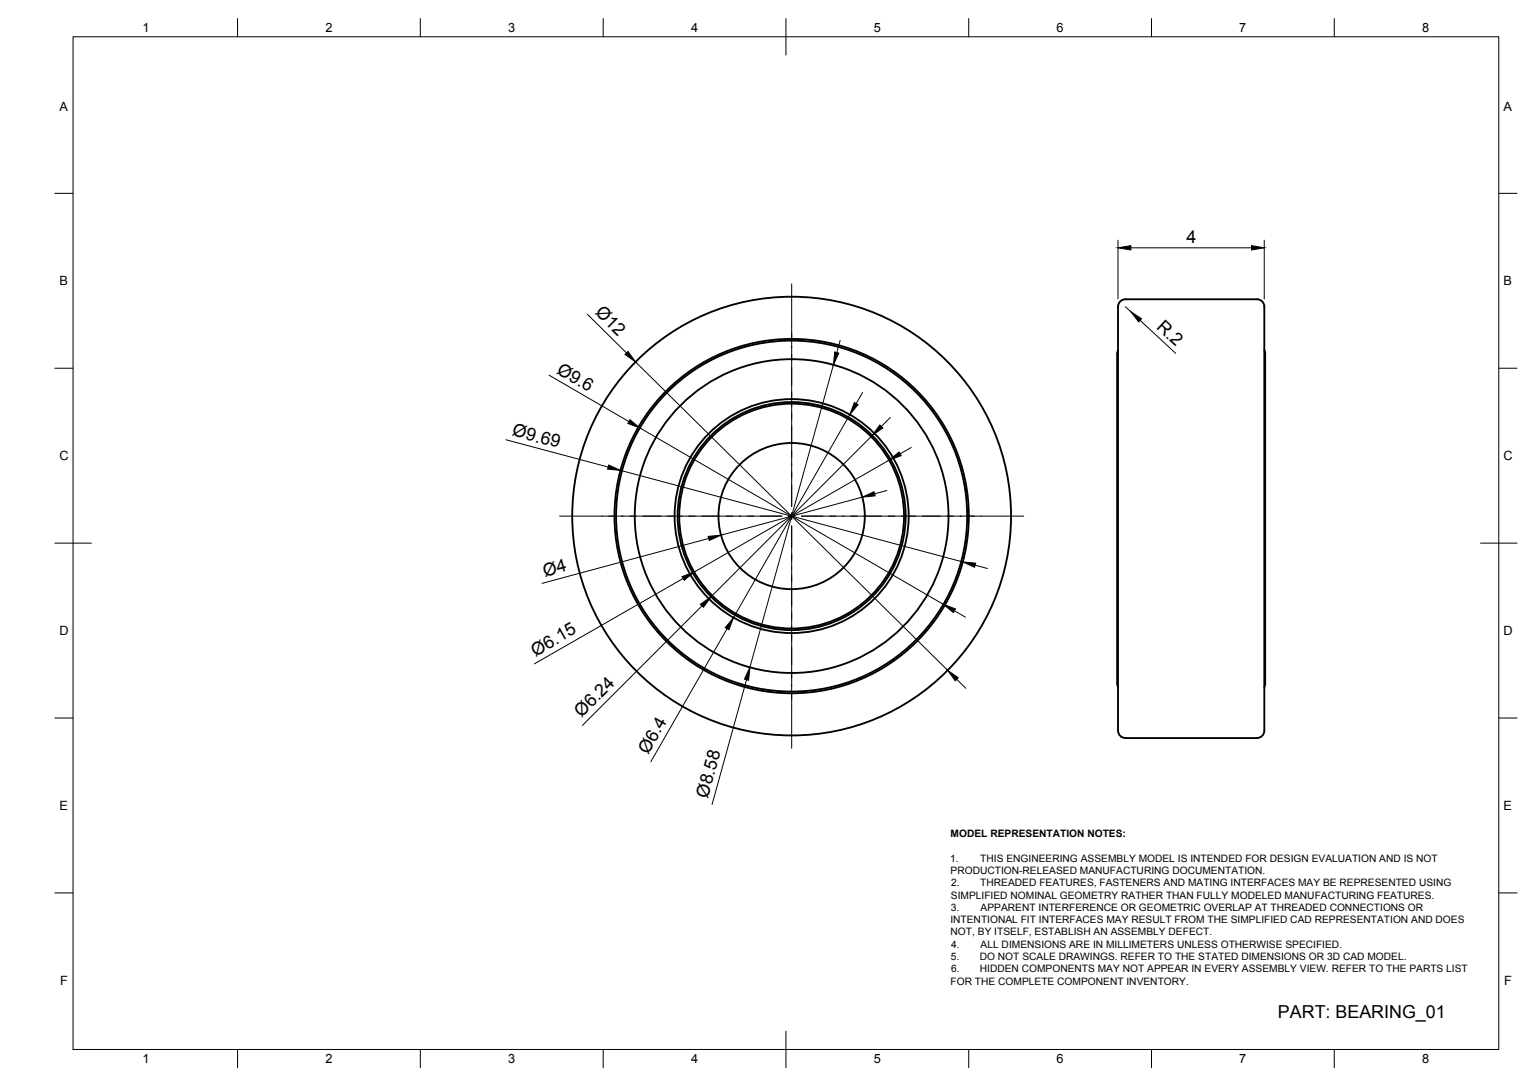
ISO-10303-21;
HEADER;
/* Generated by software containing ST-Developer
 * from STEP Tools, Inc. (www.steptools.com) 
 */

FILE_DESCRIPTION(
/* description */ (''),
/* implementation_level */ '2;1');

FILE_NAME(
/* name */ 'Bearing_01.step',
/* time_stamp */ '2026-10-04T15:18:51-07:00',
/* author */ (''),
/* organization */ (''),
/* preprocessor_version */ 'ST-DEVELOPER v20.2',
/* originating_system */ 'Autodesk Translation Framework v15.15.0.0',
/* authorisation */ '');

FILE_SCHEMA (('AUTOMOTIVE_DESIGN { 1 0 10303 214 3 1 1 }'));
ENDSEC;

DATA;
#10=MECHANICAL_DESIGN_GEOMETRIC_PRESENTATION_REPRESENTATION('',(#68,#69,#70,#71),#9891);
#52=SHAPE_REPRESENTATION_RELATIONSHIP('SRR','None',#9923,#60);
#60=ADVANCED_BREP_SHAPE_REPRESENTATION('',(#82,#83,#84,#85),#9883);
#68=STYLED_ITEM('',(#9972),#82);
#69=STYLED_ITEM('',(#9972),#83);
#70=STYLED_ITEM('',(#9972),#84);
#71=STYLED_ITEM('',(#9972),#85);
#82=MANIFOLD_SOLID_BREP('Body1',#5616);
#83=MANIFOLD_SOLID_BREP('Body2',#5617);
#84=MANIFOLD_SOLID_BREP('Body3',#5618);
#85=MANIFOLD_SOLID_BREP('Body4',#5619);
#96=FACE_BOUND('',#746,.T.);
#97=FACE_BOUND('',#748,.T.);
#98=FACE_BOUND('',#750,.T.);
#99=FACE_BOUND('',#752,.T.);
#100=FACE_BOUND('',#764,.T.);
#101=FACE_BOUND('',#766,.T.);
#102=FACE_BOUND('',#768,.T.);
#103=FACE_BOUND('',#770,.T.);
#104=FACE_BOUND('',#784,.T.);
#105=FACE_BOUND('',#786,.T.);
#106=FACE_BOUND('',#788,.T.);
#107=FACE_BOUND('',#790,.T.);
#108=FACE_BOUND('',#792,.T.);
#109=FACE_BOUND('',#806,.T.);
#110=FACE_BOUND('',#808,.T.);
#111=FACE_BOUND('',#810,.T.);
#112=FACE_BOUND('',#812,.T.);
#113=FACE_BOUND('',#814,.T.);
#161=PLANE('',#5744);
#162=PLANE('',#5745);
#163=PLANE('',#5746);
#164=PLANE('',#5747);
#165=PLANE('',#5777);
#166=PLANE('',#5778);
#167=PLANE('',#5779);
#168=PLANE('',#5780);
#169=PLANE('',#5817);
#170=PLANE('',#5818);
#171=PLANE('',#5819);
#172=PLANE('',#5820);
#173=PLANE('',#5821);
#174=PLANE('',#5858);
#175=PLANE('',#5859);
#176=PLANE('',#5860);
#177=PLANE('',#5861);
#178=PLANE('',#5862);
#337=TOROIDAL_SURFACE('',#5733,5.8,0.2);
#338=TOROIDAL_SURFACE('',#5739,5.8,0.2);
#339=TOROIDAL_SURFACE('',#5754,3.25741379310345,0.138976293103448);
#340=TOROIDAL_SURFACE('',#5760,3.25741379310345,0.138976293103448);
#341=TOROIDAL_SURFACE('',#5768,2.2,0.2);
#342=TOROIDAL_SURFACE('',#5774,2.2,0.2);
#343=TOROIDAL_SURFACE('',#5784,4.14313829631318,0.0900000000000005);
#344=TOROIDAL_SURFACE('',#5790,4.38370090847553,0.0200000000000002);
#345=TOROIDAL_SURFACE('',#5793,4.58,0.119999999999999);
#346=TOROIDAL_SURFACE('',#5799,4.51071796769724,0.12);
#347=TOROIDAL_SURFACE('',#5802,4.51071796769724,0.22);
#348=TOROIDAL_SURFACE('',#5808,4.58,0.219999999999999);
#349=TOROIDAL_SURFACE('',#5811,4.38370090847553,0.12);
#350=TOROIDAL_SURFACE('',#5825,4.14313829631318,0.0900000000000005);
#351=TOROIDAL_SURFACE('',#5831,4.38370090847553,0.0200000000000002);
#352=TOROIDAL_SURFACE('',#5834,4.58,0.119999999999999);
#353=TOROIDAL_SURFACE('',#5840,4.51071796769724,0.12);
#354=TOROIDAL_SURFACE('',#5843,4.51071796769724,0.22);
#355=TOROIDAL_SURFACE('',#5849,4.58,0.219999999999999);
#356=TOROIDAL_SURFACE('',#5852,4.38370090847553,0.12);
#380=CONICAL_SURFACE('',#5731,4.8,0.785398163397444);
#381=CONICAL_SURFACE('',#5742,4.845,0.785398163397444);
#382=CONICAL_SURFACE('',#5748,3.1184375,0.785398163397448);
#383=CONICAL_SURFACE('',#5766,3.0734375,0.785398163397448);
#384=CONICAL_SURFACE('',#5788,4.36638040039984,0.52359877559829);
#385=CONICAL_SURFACE('',#5797,4.57071796769724,1.04719755119659);
#386=CONICAL_SURFACE('',#5806,4.62071796769724,1.04719755119659);
#387=CONICAL_SURFACE('',#5815,4.27977786002139,0.52359877559829);
#388=CONICAL_SURFACE('',#5829,4.36638040039984,0.52359877559829);
#389=CONICAL_SURFACE('',#5838,4.57071796769724,1.04719755119659);
#390=CONICAL_SURFACE('',#5847,4.62071796769724,1.04719755119659);
#391=CONICAL_SURFACE('',#5856,4.27977786002139,0.52359877559829);
#407=FACE_OUTER_BOUND('',#737,.T.);
#408=FACE_OUTER_BOUND('',#738,.T.);
#409=FACE_OUTER_BOUND('',#739,.T.);
#410=FACE_OUTER_BOUND('',#740,.T.);
#411=FACE_OUTER_BOUND('',#741,.T.);
#412=FACE_OUTER_BOUND('',#742,.T.);
#413=FACE_OUTER_BOUND('',#743,.T.);
#414=FACE_OUTER_BOUND('',#744,.T.);
#415=FACE_OUTER_BOUND('',#745,.T.);
#416=FACE_OUTER_BOUND('',#747,.T.);
#417=FACE_OUTER_BOUND('',#749,.T.);
#418=FACE_OUTER_BOUND('',#751,.T.);
#419=FACE_OUTER_BOUND('',#753,.T.);
#420=FACE_OUTER_BOUND('',#754,.T.);
#421=FACE_OUTER_BOUND('',#755,.T.);
#422=FACE_OUTER_BOUND('',#756,.T.);
#423=FACE_OUTER_BOUND('',#757,.T.);
#424=FACE_OUTER_BOUND('',#758,.T.);
#425=FACE_OUTER_BOUND('',#759,.T.);
#426=FACE_OUTER_BOUND('',#760,.T.);
#427=FACE_OUTER_BOUND('',#761,.T.);
#428=FACE_OUTER_BOUND('',#762,.T.);
#429=FACE_OUTER_BOUND('',#763,.T.);
#430=FACE_OUTER_BOUND('',#765,.T.);
#431=FACE_OUTER_BOUND('',#767,.T.);
#432=FACE_OUTER_BOUND('',#769,.T.);
#433=FACE_OUTER_BOUND('',#771,.T.);
#434=FACE_OUTER_BOUND('',#772,.T.);
#435=FACE_OUTER_BOUND('',#773,.T.);
#436=FACE_OUTER_BOUND('',#774,.T.);
#437=FACE_OUTER_BOUND('',#775,.T.);
#438=FACE_OUTER_BOUND('',#776,.T.);
#439=FACE_OUTER_BOUND('',#777,.T.);
#440=FACE_OUTER_BOUND('',#778,.T.);
#441=FACE_OUTER_BOUND('',#779,.T.);
#442=FACE_OUTER_BOUND('',#780,.T.);
#443=FACE_OUTER_BOUND('',#781,.T.);
#444=FACE_OUTER_BOUND('',#782,.T.);
#445=FACE_OUTER_BOUND('',#783,.T.);
#446=FACE_OUTER_BOUND('',#785,.T.);
#447=FACE_OUTER_BOUND('',#787,.T.);
#448=FACE_OUTER_BOUND('',#789,.T.);
#449=FACE_OUTER_BOUND('',#791,.T.);
#450=FACE_OUTER_BOUND('',#793,.T.);
#451=FACE_OUTER_BOUND('',#794,.T.);
#452=FACE_OUTER_BOUND('',#795,.T.);
#453=FACE_OUTER_BOUND('',#796,.T.);
#454=FACE_OUTER_BOUND('',#797,.T.);
#455=FACE_OUTER_BOUND('',#798,.T.);
#456=FACE_OUTER_BOUND('',#799,.T.);
#457=FACE_OUTER_BOUND('',#800,.T.);
#458=FACE_OUTER_BOUND('',#801,.T.);
#459=FACE_OUTER_BOUND('',#802,.T.);
#460=FACE_OUTER_BOUND('',#803,.T.);
#461=FACE_OUTER_BOUND('',#804,.T.);
#462=FACE_OUTER_BOUND('',#805,.T.);
#463=FACE_OUTER_BOUND('',#807,.T.);
#464=FACE_OUTER_BOUND('',#809,.T.);
#465=FACE_OUTER_BOUND('',#811,.T.);
#466=FACE_OUTER_BOUND('',#813,.T.);
#737=EDGE_LOOP('',(#3646,#3647,#3648,#3649));
#738=EDGE_LOOP('',(#3650,#3651,#3652,#3653));
#739=EDGE_LOOP('',(#3654,#3655,#3656,#3657,#3658));
#740=EDGE_LOOP('',(#3659,#3660,#3661,#3662,#3663));
#741=EDGE_LOOP('',(#3664,#3665,#3666,#3667));
#742=EDGE_LOOP('',(#3668,#3669,#3670,#3671));
#743=EDGE_LOOP('',(#3672,#3673,#3674,#3675));
#744=EDGE_LOOP('',(#3676,#3677,#3678,#3679));
#745=EDGE_LOOP('',(#3680));
#746=EDGE_LOOP('',(#3681));
#747=EDGE_LOOP('',(#3682));
#748=EDGE_LOOP('',(#3683));
#749=EDGE_LOOP('',(#3684));
#750=EDGE_LOOP('',(#3685));
#751=EDGE_LOOP('',(#3686));
#752=EDGE_LOOP('',(#3687));
#753=EDGE_LOOP('',(#3688,#3689,#3690,#3691,#3692));
#754=EDGE_LOOP('',(#3693,#3694,#3695,#3696,#3697));
#755=EDGE_LOOP('',(#3698,#3699,#3700,#3701));
#756=EDGE_LOOP('',(#3702,#3703,#3704,#3705));
#757=EDGE_LOOP('',(#3706,#3707,#3708,#3709));
#758=EDGE_LOOP('',(#3710,#3711,#3712,#3713));
#759=EDGE_LOOP('',(#3714,#3715,#3716,#3717));
#760=EDGE_LOOP('',(#3718,#3719,#3720,#3721));
#761=EDGE_LOOP('',(#3722,#3723,#3724,#3725));
#762=EDGE_LOOP('',(#3726,#3727,#3728,#3729));
#763=EDGE_LOOP('',(#3730));
#764=EDGE_LOOP('',(#3731));
#765=EDGE_LOOP('',(#3732));
#766=EDGE_LOOP('',(#3733));
#767=EDGE_LOOP('',(#3734));
#768=EDGE_LOOP('',(#3735));
#769=EDGE_LOOP('',(#3736));
#770=EDGE_LOOP('',(#3737));
#771=EDGE_LOOP('',(#3738,#3739,#3740,#3741));
#772=EDGE_LOOP('',(#3742,#3743,#3744,#3745));
#773=EDGE_LOOP('',(#3746,#3747,#3748,#3749));
#774=EDGE_LOOP('',(#3750,#3751,#3752,#3753));
#775=EDGE_LOOP('',(#3754,#3755,#3756,#3757));
#776=EDGE_LOOP('',(#3758,#3759,#3760,#3761));
#777=EDGE_LOOP('',(#3762,#3763,#3764,#3765));
#778=EDGE_LOOP('',(#3766,#3767,#3768,#3769));
#779=EDGE_LOOP('',(#3770,#3771,#3772,#3773));
#780=EDGE_LOOP('',(#3774,#3775,#3776,#3777));
#781=EDGE_LOOP('',(#3778,#3779,#3780,#3781));
#782=EDGE_LOOP('',(#3782,#3783,#3784,#3785));
#783=EDGE_LOOP('',(#3786));
#784=EDGE_LOOP('',(#3787));
#785=EDGE_LOOP('',(#3788));
#786=EDGE_LOOP('',(#3789));
#787=EDGE_LOOP('',(#3790));
#788=EDGE_LOOP('',(#3791));
#789=EDGE_LOOP('',(#3792));
#790=EDGE_LOOP('',(#3793));
#791=EDGE_LOOP('',(#3794));
#792=EDGE_LOOP('',(#3795));
#793=EDGE_LOOP('',(#3796,#3797,#3798,#3799));
#794=EDGE_LOOP('',(#3800,#3801,#3802,#3803));
#795=EDGE_LOOP('',(#3804,#3805,#3806,#3807));
#796=EDGE_LOOP('',(#3808,#3809,#3810,#3811));
#797=EDGE_LOOP('',(#3812,#3813,#3814,#3815));
#798=EDGE_LOOP('',(#3816,#3817,#3818,#3819));
#799=EDGE_LOOP('',(#3820,#3821,#3822,#3823));
#800=EDGE_LOOP('',(#3824,#3825,#3826,#3827));
#801=EDGE_LOOP('',(#3828,#3829,#3830,#3831));
#802=EDGE_LOOP('',(#3832,#3833,#3834,#3835));
#803=EDGE_LOOP('',(#3836,#3837,#3838,#3839));
#804=EDGE_LOOP('',(#3840,#3841,#3842,#3843));
#805=EDGE_LOOP('',(#3844));
#806=EDGE_LOOP('',(#3845));
#807=EDGE_LOOP('',(#3846));
#808=EDGE_LOOP('',(#3847));
#809=EDGE_LOOP('',(#3848));
#810=EDGE_LOOP('',(#3849));
#811=EDGE_LOOP('',(#3850));
#812=EDGE_LOOP('',(#3851));
#813=EDGE_LOOP('',(#3852));
#814=EDGE_LOOP('',(#3853));
#1132=LINE('',#8145,#1596);
#1133=LINE('',#8151,#1597);
#1134=LINE('',#8159,#1598);
#1135=LINE('',#8163,#1599);
#1136=LINE('',#8174,#1600);
#1137=LINE('',#8181,#1601);
#1138=LINE('',#8192,#1602);
#1139=LINE('',#8197,#1603);
#1140=LINE('',#8207,#1604);
#1141=LINE('',#8217,#1605);
#1142=LINE('',#8221,#1606);
#1143=LINE('',#8231,#1607);
#1144=LINE('',#8245,#1608);
#1145=LINE('',#8256,#1609);
#1146=LINE('',#8270,#1610);
#1147=LINE('',#8284,#1611);
#1148=LINE('',#8298,#1612);
#1149=LINE('',#8308,#1613);
#1150=LINE('',#8319,#1614);
#1151=LINE('',#8333,#1615);
#1152=LINE('',#8347,#1616);
#1153=LINE('',#8361,#1617);
#1596=VECTOR('',#6379,4.8);
#1597=VECTOR('',#6386,4.872);
#1598=VECTOR('',#6395,4.8);
#1599=VECTOR('',#6400,4.8);
#1600=VECTOR('',#6415,6.);
#1601=VECTOR('',#6424,4.845);
#1602=VECTOR('',#6439,3.1184375);
#1603=VECTOR('',#6446,3.1184375);
#1604=VECTOR('',#6459,3.272);
#1605=VECTOR('',#6472,3.1184375);
#1606=VECTOR('',#6477,3.0734375);
#1607=VECTOR('',#6490,2.);
#1608=VECTOR('',#6511,3.2);
#1609=VECTOR('',#6526,4.36638040039984);
#1610=VECTOR('',#6545,4.57071796769724);
#1611=VECTOR('',#6564,4.62071796769724);
#1612=VECTOR('',#6583,4.27977786002139);
#1613=VECTOR('',#6598,3.2);
#1614=VECTOR('',#6613,4.36638040039984);
#1615=VECTOR('',#6632,4.57071796769724);
#1616=VECTOR('',#6651,4.62071796769724);
#1617=VECTOR('',#6670,4.27977786002139);
#2060=CIRCLE('',#5722,4.8);
#2061=CIRCLE('',#5723,4.8);
#2062=CIRCLE('',#5725,4.872);
#2063=CIRCLE('',#5726,4.872);
#2064=CIRCLE('',#5728,4.8);
#2065=CIRCLE('',#5729,4.8);
#2066=CIRCLE('',#5730,4.8);
#2067=CIRCLE('',#5732,4.845);
#2068=CIRCLE('',#5734,6.);
#2069=CIRCLE('',#5735,0.2);
#2070=CIRCLE('',#5736,5.8);
#2071=CIRCLE('',#5738,6.);
#2072=CIRCLE('',#5740,5.8);
#2073=CIRCLE('',#5741,0.2);
#2074=CIRCLE('',#5743,4.845);
#2075=CIRCLE('',#5749,3.1184375);
#2076=CIRCLE('',#5750,3.0734375);
#2077=CIRCLE('',#5751,3.1184375);
#2078=CIRCLE('',#5753,3.1184375);
#2079=CIRCLE('',#5755,0.138976293103448);
#2080=CIRCLE('',#5756,3.2);
#2081=CIRCLE('',#5758,3.272);
#2082=CIRCLE('',#5759,3.272);
#2083=CIRCLE('',#5761,3.2);
#2084=CIRCLE('',#5762,0.138976293103448);
#2085=CIRCLE('',#5763,3.1184375);
#2086=CIRCLE('',#5765,3.1184375);
#2087=CIRCLE('',#5767,3.0734375);
#2088=CIRCLE('',#5769,2.2);
#2089=CIRCLE('',#5770,0.2);
#2090=CIRCLE('',#5771,2.);
#2091=CIRCLE('',#5773,2.);
#2092=CIRCLE('',#5775,0.2);
#2093=CIRCLE('',#5776,2.2);
#2094=CIRCLE('',#5782,3.2);
#2095=CIRCLE('',#5783,3.2);
#2096=CIRCLE('',#5785,4.22108058265378);
#2097=CIRCLE('',#5786,0.0900000000000005);
#2098=CIRCLE('',#5787,4.14313829631318);
#2099=CIRCLE('',#5789,4.36638040039984);
#2100=CIRCLE('',#5791,4.38370090847553);
#2101=CIRCLE('',#5792,0.0200000000000002);
#2102=CIRCLE('',#5794,4.64);
#2103=CIRCLE('',#5795,0.119999999999999);
#2104=CIRCLE('',#5796,4.58);
#2105=CIRCLE('',#5798,4.57071796769724);
#2106=CIRCLE('',#5800,4.39071796769724);
#2107=CIRCLE('',#5801,0.12);
#2108=CIRCLE('',#5803,4.62071796769724);
#2109=CIRCLE('',#5804,0.22);
#2110=CIRCLE('',#5805,4.29071796769724);
#2111=CIRCLE('',#5807,4.69);
#2112=CIRCLE('',#5809,4.58);
#2113=CIRCLE('',#5810,0.219999999999999);
#2114=CIRCLE('',#5812,4.27977786002139);
#2115=CIRCLE('',#5813,0.12);
#2116=CIRCLE('',#5814,4.38370090847553);
#2117=CIRCLE('',#5816,4.13736479362129);
#2118=CIRCLE('',#5823,3.2);
#2119=CIRCLE('',#5824,3.2);
#2120=CIRCLE('',#5826,4.22108058265378);
#2121=CIRCLE('',#5827,0.0900000000000005);
#2122=CIRCLE('',#5828,4.14313829631318);
#2123=CIRCLE('',#5830,4.36638040039984);
#2124=CIRCLE('',#5832,4.38370090847553);
#2125=CIRCLE('',#5833,0.0200000000000002);
#2126=CIRCLE('',#5835,4.64);
#2127=CIRCLE('',#5836,0.119999999999999);
#2128=CIRCLE('',#5837,4.58);
#2129=CIRCLE('',#5839,4.57071796769724);
#2130=CIRCLE('',#5841,4.39071796769724);
#2131=CIRCLE('',#5842,0.12);
#2132=CIRCLE('',#5844,4.62071796769724);
#2133=CIRCLE('',#5845,0.22);
#2134=CIRCLE('',#5846,4.29071796769724);
#2135=CIRCLE('',#5848,4.69);
#2136=CIRCLE('',#5850,4.58);
#2137=CIRCLE('',#5851,0.219999999999999);
#2138=CIRCLE('',#5853,4.27977786002139);
#2139=CIRCLE('',#5854,0.12);
#2140=CIRCLE('',#5855,4.38370090847553);
#2141=CIRCLE('',#5857,4.13736479362129);
#2365=VERTEX_POINT('',#8142);
#2366=VERTEX_POINT('',#8144);
#2367=VERTEX_POINT('',#8148);
#2368=VERTEX_POINT('',#8150);
#2369=VERTEX_POINT('',#8154);
#2370=VERTEX_POINT('',#8155);
#2371=VERTEX_POINT('',#8158);
#2372=VERTEX_POINT('',#8162);
#2373=VERTEX_POINT('',#8166);
#2374=VERTEX_POINT('',#8168);
#2375=VERTEX_POINT('',#8172);
#2376=VERTEX_POINT('',#8176);
#2377=VERTEX_POINT('',#8180);
#2378=VERTEX_POINT('',#8188);
#2379=VERTEX_POINT('',#8189);
#2380=VERTEX_POINT('',#8191);
#2381=VERTEX_POINT('',#8196);
#2382=VERTEX_POINT('',#8200);
#2383=VERTEX_POINT('',#8204);
#2384=VERTEX_POINT('',#8206);
#2385=VERTEX_POINT('',#8210);
#2386=VERTEX_POINT('',#8212);
#2387=VERTEX_POINT('',#8216);
#2388=VERTEX_POINT('',#8220);
#2389=VERTEX_POINT('',#8224);
#2390=VERTEX_POINT('',#8226);
#2391=VERTEX_POINT('',#8230);
#2392=VERTEX_POINT('',#8234);
#2393=VERTEX_POINT('',#8242);
#2394=VERTEX_POINT('',#8244);
#2395=VERTEX_POINT('',#8248);
#2396=VERTEX_POINT('',#8250);
#2397=VERTEX_POINT('',#8254);
#2398=VERTEX_POINT('',#8258);
#2399=VERTEX_POINT('',#8262);
#2400=VERTEX_POINT('',#8264);
#2401=VERTEX_POINT('',#8268);
#2402=VERTEX_POINT('',#8272);
#2403=VERTEX_POINT('',#8276);
#2404=VERTEX_POINT('',#8278);
#2405=VERTEX_POINT('',#8282);
#2406=VERTEX_POINT('',#8286);
#2407=VERTEX_POINT('',#8290);
#2408=VERTEX_POINT('',#8292);
#2409=VERTEX_POINT('',#8296);
#2410=VERTEX_POINT('',#8305);
#2411=VERTEX_POINT('',#8307);
#2412=VERTEX_POINT('',#8311);
#2413=VERTEX_POINT('',#8313);
#2414=VERTEX_POINT('',#8317);
#2415=VERTEX_POINT('',#8321);
#2416=VERTEX_POINT('',#8325);
#2417=VERTEX_POINT('',#8327);
#2418=VERTEX_POINT('',#8331);
#2419=VERTEX_POINT('',#8335);
#2420=VERTEX_POINT('',#8339);
#2421=VERTEX_POINT('',#8341);
#2422=VERTEX_POINT('',#8345);
#2423=VERTEX_POINT('',#8349);
#2424=VERTEX_POINT('',#8353);
#2425=VERTEX_POINT('',#8355);
#2426=VERTEX_POINT('',#8359);
#2868=EDGE_CURVE('',#2365,#2365,#2060,.T.);
#2869=EDGE_CURVE('',#2365,#2366,#1132,.T.);
#2870=EDGE_CURVE('',#2366,#2366,#2061,.T.);
#2871=EDGE_CURVE('',#2367,#2367,#2062,.T.);
#2872=EDGE_CURVE('',#2367,#2368,#1133,.T.);
#2873=EDGE_CURVE('',#2368,#2368,#2063,.T.);
#2874=EDGE_CURVE('',#2369,#2370,#2064,.T.);
#2875=EDGE_CURVE('',#2370,#2369,#2065,.T.);
#2876=EDGE_CURVE('',#2370,#2371,#1134,.T.);
#2877=EDGE_CURVE('',#2371,#2371,#2066,.T.);
#2878=EDGE_CURVE('',#2369,#2372,#1135,.T.);
#2879=EDGE_CURVE('',#2372,#2372,#2067,.T.);
#2880=EDGE_CURVE('',#2373,#2373,#2068,.T.);
#2881=EDGE_CURVE('',#2373,#2374,#2069,.T.);
#2882=EDGE_CURVE('',#2374,#2374,#2070,.T.);
#2883=EDGE_CURVE('',#2375,#2375,#2071,.T.);
#2884=EDGE_CURVE('',#2375,#2373,#1136,.T.);
#2885=EDGE_CURVE('',#2376,#2376,#2072,.T.);
#2886=EDGE_CURVE('',#2376,#2375,#2073,.T.);
#2887=EDGE_CURVE('',#2366,#2377,#1137,.T.);
#2888=EDGE_CURVE('',#2377,#2377,#2074,.T.);
#2889=EDGE_CURVE('',#2378,#2379,#2075,.T.);
#2890=EDGE_CURVE('',#2379,#2380,#1138,.T.);
#2891=EDGE_CURVE('',#2380,#2380,#2076,.T.);
#2892=EDGE_CURVE('',#2379,#2378,#2077,.T.);
#2893=EDGE_CURVE('',#2378,#2381,#1139,.T.);
#2894=EDGE_CURVE('',#2381,#2381,#2078,.T.);
#2895=EDGE_CURVE('',#2381,#2382,#2079,.T.);
#2896=EDGE_CURVE('',#2382,#2382,#2080,.T.);
#2897=EDGE_CURVE('',#2383,#2383,#2081,.T.);
#2898=EDGE_CURVE('',#2383,#2384,#1140,.T.);
#2899=EDGE_CURVE('',#2384,#2384,#2082,.T.);
#2900=EDGE_CURVE('',#2385,#2385,#2083,.T.);
#2901=EDGE_CURVE('',#2385,#2386,#2084,.T.);
#2902=EDGE_CURVE('',#2386,#2386,#2085,.T.);
#2903=EDGE_CURVE('',#2386,#2387,#1141,.T.);
#2904=EDGE_CURVE('',#2387,#2387,#2086,.T.);
#2905=EDGE_CURVE('',#2387,#2388,#1142,.T.);
#2906=EDGE_CURVE('',#2388,#2388,#2087,.T.);
#2907=EDGE_CURVE('',#2389,#2389,#2088,.T.);
#2908=EDGE_CURVE('',#2389,#2390,#2089,.T.);
#2909=EDGE_CURVE('',#2390,#2390,#2090,.T.);
#2910=EDGE_CURVE('',#2390,#2391,#1143,.T.);
#2911=EDGE_CURVE('',#2391,#2391,#2091,.T.);
#2912=EDGE_CURVE('',#2391,#2392,#2092,.T.);
#2913=EDGE_CURVE('',#2392,#2392,#2093,.T.);
#2914=EDGE_CURVE('',#2393,#2393,#2094,.T.);
#2915=EDGE_CURVE('',#2393,#2394,#1144,.T.);
#2916=EDGE_CURVE('',#2394,#2394,#2095,.T.);
#2917=EDGE_CURVE('',#2395,#2395,#2096,.T.);
#2918=EDGE_CURVE('',#2395,#2396,#2097,.T.);
#2919=EDGE_CURVE('',#2396,#2396,#2098,.T.);
#2920=EDGE_CURVE('',#2397,#2397,#2099,.T.);
#2921=EDGE_CURVE('',#2397,#2395,#1145,.T.);
#2922=EDGE_CURVE('',#2398,#2398,#2100,.T.);
#2923=EDGE_CURVE('',#2398,#2397,#2101,.T.);
#2924=EDGE_CURVE('',#2399,#2399,#2102,.T.);
#2925=EDGE_CURVE('',#2399,#2400,#2103,.T.);
#2926=EDGE_CURVE('',#2400,#2400,#2104,.T.);
#2927=EDGE_CURVE('',#2401,#2401,#2105,.T.);
#2928=EDGE_CURVE('',#2401,#2399,#1146,.T.);
#2929=EDGE_CURVE('',#2402,#2402,#2106,.T.);
#2930=EDGE_CURVE('',#2402,#2401,#2107,.T.);
#2931=EDGE_CURVE('',#2403,#2403,#2108,.T.);
#2932=EDGE_CURVE('',#2403,#2404,#2109,.T.);
#2933=EDGE_CURVE('',#2404,#2404,#2110,.T.);
#2934=EDGE_CURVE('',#2405,#2405,#2111,.T.);
#2935=EDGE_CURVE('',#2405,#2403,#1147,.T.);
#2936=EDGE_CURVE('',#2406,#2406,#2112,.T.);
#2937=EDGE_CURVE('',#2406,#2405,#2113,.T.);
#2938=EDGE_CURVE('',#2407,#2407,#2114,.T.);
#2939=EDGE_CURVE('',#2407,#2408,#2115,.T.);
#2940=EDGE_CURVE('',#2408,#2408,#2116,.T.);
#2941=EDGE_CURVE('',#2409,#2409,#2117,.T.);
#2942=EDGE_CURVE('',#2409,#2407,#1148,.T.);
#2943=EDGE_CURVE('',#2410,#2410,#2118,.T.);
#2944=EDGE_CURVE('',#2410,#2411,#1149,.T.);
#2945=EDGE_CURVE('',#2411,#2411,#2119,.T.);
#2946=EDGE_CURVE('',#2412,#2412,#2120,.T.);
#2947=EDGE_CURVE('',#2412,#2413,#2121,.T.);
#2948=EDGE_CURVE('',#2413,#2413,#2122,.T.);
#2949=EDGE_CURVE('',#2414,#2414,#2123,.T.);
#2950=EDGE_CURVE('',#2414,#2412,#1150,.T.);
#2951=EDGE_CURVE('',#2415,#2415,#2124,.T.);
#2952=EDGE_CURVE('',#2415,#2414,#2125,.T.);
#2953=EDGE_CURVE('',#2416,#2416,#2126,.T.);
#2954=EDGE_CURVE('',#2416,#2417,#2127,.T.);
#2955=EDGE_CURVE('',#2417,#2417,#2128,.T.);
#2956=EDGE_CURVE('',#2418,#2418,#2129,.T.);
#2957=EDGE_CURVE('',#2418,#2416,#1151,.T.);
#2958=EDGE_CURVE('',#2419,#2419,#2130,.T.);
#2959=EDGE_CURVE('',#2419,#2418,#2131,.T.);
#2960=EDGE_CURVE('',#2420,#2420,#2132,.T.);
#2961=EDGE_CURVE('',#2420,#2421,#2133,.T.);
#2962=EDGE_CURVE('',#2421,#2421,#2134,.T.);
#2963=EDGE_CURVE('',#2422,#2422,#2135,.T.);
#2964=EDGE_CURVE('',#2422,#2420,#1152,.T.);
#2965=EDGE_CURVE('',#2423,#2423,#2136,.T.);
#2966=EDGE_CURVE('',#2423,#2422,#2137,.T.);
#2967=EDGE_CURVE('',#2424,#2424,#2138,.T.);
#2968=EDGE_CURVE('',#2424,#2425,#2139,.T.);
#2969=EDGE_CURVE('',#2425,#2425,#2140,.T.);
#2970=EDGE_CURVE('',#2426,#2426,#2141,.T.);
#2971=EDGE_CURVE('',#2426,#2424,#1153,.T.);
#3646=ORIENTED_EDGE('',*,*,#2868,.F.);
#3647=ORIENTED_EDGE('',*,*,#2869,.T.);
#3648=ORIENTED_EDGE('',*,*,#2870,.T.);
#3649=ORIENTED_EDGE('',*,*,#2869,.F.);
#3650=ORIENTED_EDGE('',*,*,#2871,.F.);
#3651=ORIENTED_EDGE('',*,*,#2872,.T.);
#3652=ORIENTED_EDGE('',*,*,#2873,.T.);
#3653=ORIENTED_EDGE('',*,*,#2872,.F.);
#3654=ORIENTED_EDGE('',*,*,#2874,.F.);
#3655=ORIENTED_EDGE('',*,*,#2875,.F.);
#3656=ORIENTED_EDGE('',*,*,#2876,.T.);
#3657=ORIENTED_EDGE('',*,*,#2877,.T.);
#3658=ORIENTED_EDGE('',*,*,#2876,.F.);
#3659=ORIENTED_EDGE('',*,*,#2874,.T.);
#3660=ORIENTED_EDGE('',*,*,#2875,.T.);
#3661=ORIENTED_EDGE('',*,*,#2878,.T.);
#3662=ORIENTED_EDGE('',*,*,#2879,.F.);
#3663=ORIENTED_EDGE('',*,*,#2878,.F.);
#3664=ORIENTED_EDGE('',*,*,#2880,.F.);
#3665=ORIENTED_EDGE('',*,*,#2881,.T.);
#3666=ORIENTED_EDGE('',*,*,#2882,.T.);
#3667=ORIENTED_EDGE('',*,*,#2881,.F.);
#3668=ORIENTED_EDGE('',*,*,#2883,.F.);
#3669=ORIENTED_EDGE('',*,*,#2884,.T.);
#3670=ORIENTED_EDGE('',*,*,#2880,.T.);
#3671=ORIENTED_EDGE('',*,*,#2884,.F.);
#3672=ORIENTED_EDGE('',*,*,#2885,.F.);
#3673=ORIENTED_EDGE('',*,*,#2886,.T.);
#3674=ORIENTED_EDGE('',*,*,#2883,.T.);
#3675=ORIENTED_EDGE('',*,*,#2886,.F.);
#3676=ORIENTED_EDGE('',*,*,#2870,.F.);
#3677=ORIENTED_EDGE('',*,*,#2887,.T.);
#3678=ORIENTED_EDGE('',*,*,#2888,.T.);
#3679=ORIENTED_EDGE('',*,*,#2887,.F.);
#3680=ORIENTED_EDGE('',*,*,#2885,.T.);
#3681=ORIENTED_EDGE('',*,*,#2888,.F.);
#3682=ORIENTED_EDGE('',*,*,#2882,.F.);
#3683=ORIENTED_EDGE('',*,*,#2879,.T.);
#3684=ORIENTED_EDGE('',*,*,#2871,.T.);
#3685=ORIENTED_EDGE('',*,*,#2877,.F.);
#3686=ORIENTED_EDGE('',*,*,#2873,.F.);
#3687=ORIENTED_EDGE('',*,*,#2868,.T.);
#3688=ORIENTED_EDGE('',*,*,#2889,.T.);
#3689=ORIENTED_EDGE('',*,*,#2890,.T.);
#3690=ORIENTED_EDGE('',*,*,#2891,.F.);
#3691=ORIENTED_EDGE('',*,*,#2890,.F.);
#3692=ORIENTED_EDGE('',*,*,#2892,.T.);
#3693=ORIENTED_EDGE('',*,*,#2889,.F.);
#3694=ORIENTED_EDGE('',*,*,#2893,.T.);
#3695=ORIENTED_EDGE('',*,*,#2894,.T.);
#3696=ORIENTED_EDGE('',*,*,#2893,.F.);
#3697=ORIENTED_EDGE('',*,*,#2892,.F.);
#3698=ORIENTED_EDGE('',*,*,#2894,.F.);
#3699=ORIENTED_EDGE('',*,*,#2895,.T.);
#3700=ORIENTED_EDGE('',*,*,#2896,.T.);
#3701=ORIENTED_EDGE('',*,*,#2895,.F.);
#3702=ORIENTED_EDGE('',*,*,#2897,.F.);
#3703=ORIENTED_EDGE('',*,*,#2898,.T.);
#3704=ORIENTED_EDGE('',*,*,#2899,.T.);
#3705=ORIENTED_EDGE('',*,*,#2898,.F.);
#3706=ORIENTED_EDGE('',*,*,#2900,.F.);
#3707=ORIENTED_EDGE('',*,*,#2901,.T.);
#3708=ORIENTED_EDGE('',*,*,#2902,.T.);
#3709=ORIENTED_EDGE('',*,*,#2901,.F.);
#3710=ORIENTED_EDGE('',*,*,#2902,.F.);
#3711=ORIENTED_EDGE('',*,*,#2903,.T.);
#3712=ORIENTED_EDGE('',*,*,#2904,.T.);
#3713=ORIENTED_EDGE('',*,*,#2903,.F.);
#3714=ORIENTED_EDGE('',*,*,#2904,.F.);
#3715=ORIENTED_EDGE('',*,*,#2905,.T.);
#3716=ORIENTED_EDGE('',*,*,#2906,.T.);
#3717=ORIENTED_EDGE('',*,*,#2905,.F.);
#3718=ORIENTED_EDGE('',*,*,#2907,.F.);
#3719=ORIENTED_EDGE('',*,*,#2908,.T.);
#3720=ORIENTED_EDGE('',*,*,#2909,.T.);
#3721=ORIENTED_EDGE('',*,*,#2908,.F.);
#3722=ORIENTED_EDGE('',*,*,#2909,.F.);
#3723=ORIENTED_EDGE('',*,*,#2910,.T.);
#3724=ORIENTED_EDGE('',*,*,#2911,.T.);
#3725=ORIENTED_EDGE('',*,*,#2910,.F.);
#3726=ORIENTED_EDGE('',*,*,#2911,.F.);
#3727=ORIENTED_EDGE('',*,*,#2912,.T.);
#3728=ORIENTED_EDGE('',*,*,#2913,.T.);
#3729=ORIENTED_EDGE('',*,*,#2912,.F.);
#3730=ORIENTED_EDGE('',*,*,#2906,.F.);
#3731=ORIENTED_EDGE('',*,*,#2907,.T.);
#3732=ORIENTED_EDGE('',*,*,#2899,.F.);
#3733=ORIENTED_EDGE('',*,*,#2900,.T.);
#3734=ORIENTED_EDGE('',*,*,#2897,.T.);
#3735=ORIENTED_EDGE('',*,*,#2896,.F.);
#3736=ORIENTED_EDGE('',*,*,#2891,.T.);
#3737=ORIENTED_EDGE('',*,*,#2913,.F.);
#3738=ORIENTED_EDGE('',*,*,#2914,.F.);
#3739=ORIENTED_EDGE('',*,*,#2915,.T.);
#3740=ORIENTED_EDGE('',*,*,#2916,.T.);
#3741=ORIENTED_EDGE('',*,*,#2915,.F.);
#3742=ORIENTED_EDGE('',*,*,#2917,.F.);
#3743=ORIENTED_EDGE('',*,*,#2918,.T.);
#3744=ORIENTED_EDGE('',*,*,#2919,.T.);
#3745=ORIENTED_EDGE('',*,*,#2918,.F.);
#3746=ORIENTED_EDGE('',*,*,#2920,.F.);
#3747=ORIENTED_EDGE('',*,*,#2921,.T.);
#3748=ORIENTED_EDGE('',*,*,#2917,.T.);
#3749=ORIENTED_EDGE('',*,*,#2921,.F.);
#3750=ORIENTED_EDGE('',*,*,#2922,.F.);
#3751=ORIENTED_EDGE('',*,*,#2923,.T.);
#3752=ORIENTED_EDGE('',*,*,#2920,.T.);
#3753=ORIENTED_EDGE('',*,*,#2923,.F.);
#3754=ORIENTED_EDGE('',*,*,#2924,.F.);
#3755=ORIENTED_EDGE('',*,*,#2925,.T.);
#3756=ORIENTED_EDGE('',*,*,#2926,.T.);
#3757=ORIENTED_EDGE('',*,*,#2925,.F.);
#3758=ORIENTED_EDGE('',*,*,#2927,.F.);
#3759=ORIENTED_EDGE('',*,*,#2928,.T.);
#3760=ORIENTED_EDGE('',*,*,#2924,.T.);
#3761=ORIENTED_EDGE('',*,*,#2928,.F.);
#3762=ORIENTED_EDGE('',*,*,#2929,.F.);
#3763=ORIENTED_EDGE('',*,*,#2930,.T.);
#3764=ORIENTED_EDGE('',*,*,#2927,.T.);
#3765=ORIENTED_EDGE('',*,*,#2930,.F.);
#3766=ORIENTED_EDGE('',*,*,#2931,.F.);
#3767=ORIENTED_EDGE('',*,*,#2932,.T.);
#3768=ORIENTED_EDGE('',*,*,#2933,.T.);
#3769=ORIENTED_EDGE('',*,*,#2932,.F.);
#3770=ORIENTED_EDGE('',*,*,#2934,.F.);
#3771=ORIENTED_EDGE('',*,*,#2935,.T.);
#3772=ORIENTED_EDGE('',*,*,#2931,.T.);
#3773=ORIENTED_EDGE('',*,*,#2935,.F.);
#3774=ORIENTED_EDGE('',*,*,#2936,.F.);
#3775=ORIENTED_EDGE('',*,*,#2937,.T.);
#3776=ORIENTED_EDGE('',*,*,#2934,.T.);
#3777=ORIENTED_EDGE('',*,*,#2937,.F.);
#3778=ORIENTED_EDGE('',*,*,#2938,.F.);
#3779=ORIENTED_EDGE('',*,*,#2939,.T.);
#3780=ORIENTED_EDGE('',*,*,#2940,.T.);
#3781=ORIENTED_EDGE('',*,*,#2939,.F.);
#3782=ORIENTED_EDGE('',*,*,#2941,.F.);
#3783=ORIENTED_EDGE('',*,*,#2942,.T.);
#3784=ORIENTED_EDGE('',*,*,#2938,.T.);
#3785=ORIENTED_EDGE('',*,*,#2942,.F.);
#3786=ORIENTED_EDGE('',*,*,#2941,.T.);
#3787=ORIENTED_EDGE('',*,*,#2916,.F.);
#3788=ORIENTED_EDGE('',*,*,#2936,.T.);
#3789=ORIENTED_EDGE('',*,*,#2940,.F.);
#3790=ORIENTED_EDGE('',*,*,#2929,.T.);
#3791=ORIENTED_EDGE('',*,*,#2933,.F.);
#3792=ORIENTED_EDGE('',*,*,#2926,.F.);
#3793=ORIENTED_EDGE('',*,*,#2922,.T.);
#3794=ORIENTED_EDGE('',*,*,#2919,.F.);
#3795=ORIENTED_EDGE('',*,*,#2914,.T.);
#3796=ORIENTED_EDGE('',*,*,#2943,.T.);
#3797=ORIENTED_EDGE('',*,*,#2944,.T.);
#3798=ORIENTED_EDGE('',*,*,#2945,.F.);
#3799=ORIENTED_EDGE('',*,*,#2944,.F.);
#3800=ORIENTED_EDGE('',*,*,#2946,.T.);
#3801=ORIENTED_EDGE('',*,*,#2947,.T.);
#3802=ORIENTED_EDGE('',*,*,#2948,.F.);
#3803=ORIENTED_EDGE('',*,*,#2947,.F.);
#3804=ORIENTED_EDGE('',*,*,#2949,.T.);
#3805=ORIENTED_EDGE('',*,*,#2950,.T.);
#3806=ORIENTED_EDGE('',*,*,#2946,.F.);
#3807=ORIENTED_EDGE('',*,*,#2950,.F.);
#3808=ORIENTED_EDGE('',*,*,#2951,.T.);
#3809=ORIENTED_EDGE('',*,*,#2952,.T.);
#3810=ORIENTED_EDGE('',*,*,#2949,.F.);
#3811=ORIENTED_EDGE('',*,*,#2952,.F.);
#3812=ORIENTED_EDGE('',*,*,#2953,.T.);
#3813=ORIENTED_EDGE('',*,*,#2954,.T.);
#3814=ORIENTED_EDGE('',*,*,#2955,.F.);
#3815=ORIENTED_EDGE('',*,*,#2954,.F.);
#3816=ORIENTED_EDGE('',*,*,#2956,.T.);
#3817=ORIENTED_EDGE('',*,*,#2957,.T.);
#3818=ORIENTED_EDGE('',*,*,#2953,.F.);
#3819=ORIENTED_EDGE('',*,*,#2957,.F.);
#3820=ORIENTED_EDGE('',*,*,#2958,.T.);
#3821=ORIENTED_EDGE('',*,*,#2959,.T.);
#3822=ORIENTED_EDGE('',*,*,#2956,.F.);
#3823=ORIENTED_EDGE('',*,*,#2959,.F.);
#3824=ORIENTED_EDGE('',*,*,#2960,.T.);
#3825=ORIENTED_EDGE('',*,*,#2961,.T.);
#3826=ORIENTED_EDGE('',*,*,#2962,.F.);
#3827=ORIENTED_EDGE('',*,*,#2961,.F.);
#3828=ORIENTED_EDGE('',*,*,#2963,.T.);
#3829=ORIENTED_EDGE('',*,*,#2964,.T.);
#3830=ORIENTED_EDGE('',*,*,#2960,.F.);
#3831=ORIENTED_EDGE('',*,*,#2964,.F.);
#3832=ORIENTED_EDGE('',*,*,#2965,.T.);
#3833=ORIENTED_EDGE('',*,*,#2966,.T.);
#3834=ORIENTED_EDGE('',*,*,#2963,.F.);
#3835=ORIENTED_EDGE('',*,*,#2966,.F.);
#3836=ORIENTED_EDGE('',*,*,#2967,.T.);
#3837=ORIENTED_EDGE('',*,*,#2968,.T.);
#3838=ORIENTED_EDGE('',*,*,#2969,.F.);
#3839=ORIENTED_EDGE('',*,*,#2968,.F.);
#3840=ORIENTED_EDGE('',*,*,#2970,.T.);
#3841=ORIENTED_EDGE('',*,*,#2971,.T.);
#3842=ORIENTED_EDGE('',*,*,#2967,.F.);
#3843=ORIENTED_EDGE('',*,*,#2971,.F.);
#3844=ORIENTED_EDGE('',*,*,#2970,.F.);
#3845=ORIENTED_EDGE('',*,*,#2945,.T.);
#3846=ORIENTED_EDGE('',*,*,#2965,.F.);
#3847=ORIENTED_EDGE('',*,*,#2969,.T.);
#3848=ORIENTED_EDGE('',*,*,#2958,.F.);
#3849=ORIENTED_EDGE('',*,*,#2962,.T.);
#3850=ORIENTED_EDGE('',*,*,#2955,.T.);
#3851=ORIENTED_EDGE('',*,*,#2951,.F.);
#3852=ORIENTED_EDGE('',*,*,#2948,.T.);
#3853=ORIENTED_EDGE('',*,*,#2943,.F.);
#5202=CYLINDRICAL_SURFACE('',#5721,4.8);
#5203=CYLINDRICAL_SURFACE('',#5724,4.872);
#5204=CYLINDRICAL_SURFACE('',#5727,4.8);
#5205=CYLINDRICAL_SURFACE('',#5737,6.);
#5206=CYLINDRICAL_SURFACE('',#5752,3.1184375);
#5207=CYLINDRICAL_SURFACE('',#5757,3.272);
#5208=CYLINDRICAL_SURFACE('',#5764,3.1184375);
#5209=CYLINDRICAL_SURFACE('',#5772,2.);
#5210=CYLINDRICAL_SURFACE('',#5781,3.2);
#5211=CYLINDRICAL_SURFACE('',#5822,3.2);
#5286=ADVANCED_FACE('',(#407),#5202,.F.);
#5287=ADVANCED_FACE('',(#408),#5203,.F.);
#5288=ADVANCED_FACE('',(#409),#5204,.F.);
#5289=ADVANCED_FACE('',(#410),#380,.F.);
#5290=ADVANCED_FACE('',(#411),#337,.T.);
#5291=ADVANCED_FACE('',(#412),#5205,.T.);
#5292=ADVANCED_FACE('',(#413),#338,.T.);
#5293=ADVANCED_FACE('',(#414),#381,.F.);
#5294=ADVANCED_FACE('',(#415,#96),#161,.F.);
#5295=ADVANCED_FACE('',(#416,#97),#162,.F.);
#5296=ADVANCED_FACE('',(#417,#98),#163,.F.);
#5297=ADVANCED_FACE('',(#418,#99),#164,.F.);
#5298=ADVANCED_FACE('',(#419),#382,.T.);
#5299=ADVANCED_FACE('',(#420),#5206,.T.);
#5300=ADVANCED_FACE('',(#421),#339,.F.);
#5301=ADVANCED_FACE('',(#422),#5207,.T.);
#5302=ADVANCED_FACE('',(#423),#340,.F.);
#5303=ADVANCED_FACE('',(#424),#5208,.T.);
#5304=ADVANCED_FACE('',(#425),#383,.T.);
#5305=ADVANCED_FACE('',(#426),#341,.T.);
#5306=ADVANCED_FACE('',(#427),#5209,.F.);
#5307=ADVANCED_FACE('',(#428),#342,.T.);
#5308=ADVANCED_FACE('',(#429,#100),#165,.F.);
#5309=ADVANCED_FACE('',(#430,#101),#166,.F.);
#5310=ADVANCED_FACE('',(#431,#102),#167,.F.);
#5311=ADVANCED_FACE('',(#432,#103),#168,.F.);
#5312=ADVANCED_FACE('',(#433),#5210,.F.);
#5313=ADVANCED_FACE('',(#434),#343,.T.);
#5314=ADVANCED_FACE('',(#435),#384,.T.);
#5315=ADVANCED_FACE('',(#436),#344,.F.);
#5316=ADVANCED_FACE('',(#437),#345,.F.);
#5317=ADVANCED_FACE('',(#438),#385,.F.);
#5318=ADVANCED_FACE('',(#439),#346,.F.);
#5319=ADVANCED_FACE('',(#440),#347,.T.);
#5320=ADVANCED_FACE('',(#441),#386,.T.);
#5321=ADVANCED_FACE('',(#442),#348,.T.);
#5322=ADVANCED_FACE('',(#443),#349,.T.);
#5323=ADVANCED_FACE('',(#444),#387,.F.);
#5324=ADVANCED_FACE('',(#445,#104),#169,.F.);
#5325=ADVANCED_FACE('',(#446,#105),#170,.F.);
#5326=ADVANCED_FACE('',(#447,#106),#171,.T.);
#5327=ADVANCED_FACE('',(#448,#107),#172,.T.);
#5328=ADVANCED_FACE('',(#449,#108),#173,.T.);
#5329=ADVANCED_FACE('',(#450),#5211,.F.);
#5330=ADVANCED_FACE('',(#451),#350,.T.);
#5331=ADVANCED_FACE('',(#452),#388,.T.);
#5332=ADVANCED_FACE('',(#453),#351,.F.);
#5333=ADVANCED_FACE('',(#454),#352,.F.);
#5334=ADVANCED_FACE('',(#455),#389,.F.);
#5335=ADVANCED_FACE('',(#456),#353,.F.);
#5336=ADVANCED_FACE('',(#457),#354,.T.);
#5337=ADVANCED_FACE('',(#458),#390,.T.);
#5338=ADVANCED_FACE('',(#459),#355,.T.);
#5339=ADVANCED_FACE('',(#460),#356,.T.);
#5340=ADVANCED_FACE('',(#461),#391,.F.);
#5341=ADVANCED_FACE('',(#462,#109),#174,.F.);
#5342=ADVANCED_FACE('',(#463,#110),#175,.F.);
#5343=ADVANCED_FACE('',(#464,#111),#176,.T.);
#5344=ADVANCED_FACE('',(#465,#112),#177,.T.);
#5345=ADVANCED_FACE('',(#466,#113),#178,.T.);
#5616=CLOSED_SHELL('',(#5286,#5287,#5288,#5289,#5290,#5291,#5292,#5293,
#5294,#5295,#5296,#5297));
#5617=CLOSED_SHELL('',(#5298,#5299,#5300,#5301,#5302,#5303,#5304,#5305,
#5306,#5307,#5308,#5309,#5310,#5311));
#5618=CLOSED_SHELL('',(#5312,#5313,#5314,#5315,#5316,#5317,#5318,#5319,
#5320,#5321,#5322,#5323,#5324,#5325,#5326,#5327,#5328));
#5619=CLOSED_SHELL('',(#5329,#5330,#5331,#5332,#5333,#5334,#5335,#5336,
#5337,#5338,#5339,#5340,#5341,#5342,#5343,#5344,#5345));
#5720=AXIS2_PLACEMENT_3D('',#8140,#6373,#6374);
#5721=AXIS2_PLACEMENT_3D('',#8141,#6375,#6376);
#5722=AXIS2_PLACEMENT_3D('',#8143,#6377,#6378);
#5723=AXIS2_PLACEMENT_3D('',#8146,#6380,#6381);
#5724=AXIS2_PLACEMENT_3D('',#8147,#6382,#6383);
#5725=AXIS2_PLACEMENT_3D('',#8149,#6384,#6385);
#5726=AXIS2_PLACEMENT_3D('',#8152,#6387,#6388);
#5727=AXIS2_PLACEMENT_3D('',#8153,#6389,#6390);
#5728=AXIS2_PLACEMENT_3D('',#8156,#6391,#6392);
#5729=AXIS2_PLACEMENT_3D('',#8157,#6393,#6394);
#5730=AXIS2_PLACEMENT_3D('',#8160,#6396,#6397);
#5731=AXIS2_PLACEMENT_3D('',#8161,#6398,#6399);
#5732=AXIS2_PLACEMENT_3D('',#8164,#6401,#6402);
#5733=AXIS2_PLACEMENT_3D('',#8165,#6403,#6404);
#5734=AXIS2_PLACEMENT_3D('',#8167,#6405,#6406);
#5735=AXIS2_PLACEMENT_3D('',#8169,#6407,#6408);
#5736=AXIS2_PLACEMENT_3D('',#8170,#6409,#6410);
#5737=AXIS2_PLACEMENT_3D('',#8171,#6411,#6412);
#5738=AXIS2_PLACEMENT_3D('',#8173,#6413,#6414);
#5739=AXIS2_PLACEMENT_3D('',#8175,#6416,#6417);
#5740=AXIS2_PLACEMENT_3D('',#8177,#6418,#6419);
#5741=AXIS2_PLACEMENT_3D('',#8178,#6420,#6421);
#5742=AXIS2_PLACEMENT_3D('',#8179,#6422,#6423);
#5743=AXIS2_PLACEMENT_3D('',#8182,#6425,#6426);
#5744=AXIS2_PLACEMENT_3D('',#8183,#6427,#6428);
#5745=AXIS2_PLACEMENT_3D('',#8184,#6429,#6430);
#5746=AXIS2_PLACEMENT_3D('',#8185,#6431,#6432);
#5747=AXIS2_PLACEMENT_3D('',#8186,#6433,#6434);
#5748=AXIS2_PLACEMENT_3D('',#8187,#6435,#6436);
#5749=AXIS2_PLACEMENT_3D('',#8190,#6437,#6438);
#5750=AXIS2_PLACEMENT_3D('',#8193,#6440,#6441);
#5751=AXIS2_PLACEMENT_3D('',#8194,#6442,#6443);
#5752=AXIS2_PLACEMENT_3D('',#8195,#6444,#6445);
#5753=AXIS2_PLACEMENT_3D('',#8198,#6447,#6448);
#5754=AXIS2_PLACEMENT_3D('',#8199,#6449,#6450);
#5755=AXIS2_PLACEMENT_3D('',#8201,#6451,#6452);
#5756=AXIS2_PLACEMENT_3D('',#8202,#6453,#6454);
#5757=AXIS2_PLACEMENT_3D('',#8203,#6455,#6456);
#5758=AXIS2_PLACEMENT_3D('',#8205,#6457,#6458);
#5759=AXIS2_PLACEMENT_3D('',#8208,#6460,#6461);
#5760=AXIS2_PLACEMENT_3D('',#8209,#6462,#6463);
#5761=AXIS2_PLACEMENT_3D('',#8211,#6464,#6465);
#5762=AXIS2_PLACEMENT_3D('',#8213,#6466,#6467);
#5763=AXIS2_PLACEMENT_3D('',#8214,#6468,#6469);
#5764=AXIS2_PLACEMENT_3D('',#8215,#6470,#6471);
#5765=AXIS2_PLACEMENT_3D('',#8218,#6473,#6474);
#5766=AXIS2_PLACEMENT_3D('',#8219,#6475,#6476);
#5767=AXIS2_PLACEMENT_3D('',#8222,#6478,#6479);
#5768=AXIS2_PLACEMENT_3D('',#8223,#6480,#6481);
#5769=AXIS2_PLACEMENT_3D('',#8225,#6482,#6483);
#5770=AXIS2_PLACEMENT_3D('',#8227,#6484,#6485);
#5771=AXIS2_PLACEMENT_3D('',#8228,#6486,#6487);
#5772=AXIS2_PLACEMENT_3D('',#8229,#6488,#6489);
#5773=AXIS2_PLACEMENT_3D('',#8232,#6491,#6492);
#5774=AXIS2_PLACEMENT_3D('',#8233,#6493,#6494);
#5775=AXIS2_PLACEMENT_3D('',#8235,#6495,#6496);
#5776=AXIS2_PLACEMENT_3D('',#8236,#6497,#6498);
#5777=AXIS2_PLACEMENT_3D('',#8237,#6499,#6500);
#5778=AXIS2_PLACEMENT_3D('',#8238,#6501,#6502);
#5779=AXIS2_PLACEMENT_3D('',#8239,#6503,#6504);
#5780=AXIS2_PLACEMENT_3D('',#8240,#6505,#6506);
#5781=AXIS2_PLACEMENT_3D('',#8241,#6507,#6508);
#5782=AXIS2_PLACEMENT_3D('',#8243,#6509,#6510);
#5783=AXIS2_PLACEMENT_3D('',#8246,#6512,#6513);
#5784=AXIS2_PLACEMENT_3D('',#8247,#6514,#6515);
#5785=AXIS2_PLACEMENT_3D('',#8249,#6516,#6517);
#5786=AXIS2_PLACEMENT_3D('',#8251,#6518,#6519);
#5787=AXIS2_PLACEMENT_3D('',#8252,#6520,#6521);
#5788=AXIS2_PLACEMENT_3D('',#8253,#6522,#6523);
#5789=AXIS2_PLACEMENT_3D('',#8255,#6524,#6525);
#5790=AXIS2_PLACEMENT_3D('',#8257,#6527,#6528);
#5791=AXIS2_PLACEMENT_3D('',#8259,#6529,#6530);
#5792=AXIS2_PLACEMENT_3D('',#8260,#6531,#6532);
#5793=AXIS2_PLACEMENT_3D('',#8261,#6533,#6534);
#5794=AXIS2_PLACEMENT_3D('',#8263,#6535,#6536);
#5795=AXIS2_PLACEMENT_3D('',#8265,#6537,#6538);
#5796=AXIS2_PLACEMENT_3D('',#8266,#6539,#6540);
#5797=AXIS2_PLACEMENT_3D('',#8267,#6541,#6542);
#5798=AXIS2_PLACEMENT_3D('',#8269,#6543,#6544);
#5799=AXIS2_PLACEMENT_3D('',#8271,#6546,#6547);
#5800=AXIS2_PLACEMENT_3D('',#8273,#6548,#6549);
#5801=AXIS2_PLACEMENT_3D('',#8274,#6550,#6551);
#5802=AXIS2_PLACEMENT_3D('',#8275,#6552,#6553);
#5803=AXIS2_PLACEMENT_3D('',#8277,#6554,#6555);
#5804=AXIS2_PLACEMENT_3D('',#8279,#6556,#6557);
#5805=AXIS2_PLACEMENT_3D('',#8280,#6558,#6559);
#5806=AXIS2_PLACEMENT_3D('',#8281,#6560,#6561);
#5807=AXIS2_PLACEMENT_3D('',#8283,#6562,#6563);
#5808=AXIS2_PLACEMENT_3D('',#8285,#6565,#6566);
#5809=AXIS2_PLACEMENT_3D('',#8287,#6567,#6568);
#5810=AXIS2_PLACEMENT_3D('',#8288,#6569,#6570);
#5811=AXIS2_PLACEMENT_3D('',#8289,#6571,#6572);
#5812=AXIS2_PLACEMENT_3D('',#8291,#6573,#6574);
#5813=AXIS2_PLACEMENT_3D('',#8293,#6575,#6576);
#5814=AXIS2_PLACEMENT_3D('',#8294,#6577,#6578);
#5815=AXIS2_PLACEMENT_3D('',#8295,#6579,#6580);
#5816=AXIS2_PLACEMENT_3D('',#8297,#6581,#6582);
#5817=AXIS2_PLACEMENT_3D('',#8299,#6584,#6585);
#5818=AXIS2_PLACEMENT_3D('',#8300,#6586,#6587);
#5819=AXIS2_PLACEMENT_3D('',#8301,#6588,#6589);
#5820=AXIS2_PLACEMENT_3D('',#8302,#6590,#6591);
#5821=AXIS2_PLACEMENT_3D('',#8303,#6592,#6593);
#5822=AXIS2_PLACEMENT_3D('',#8304,#6594,#6595);
#5823=AXIS2_PLACEMENT_3D('',#8306,#6596,#6597);
#5824=AXIS2_PLACEMENT_3D('',#8309,#6599,#6600);
#5825=AXIS2_PLACEMENT_3D('',#8310,#6601,#6602);
#5826=AXIS2_PLACEMENT_3D('',#8312,#6603,#6604);
#5827=AXIS2_PLACEMENT_3D('',#8314,#6605,#6606);
#5828=AXIS2_PLACEMENT_3D('',#8315,#6607,#6608);
#5829=AXIS2_PLACEMENT_3D('',#8316,#6609,#6610);
#5830=AXIS2_PLACEMENT_3D('',#8318,#6611,#6612);
#5831=AXIS2_PLACEMENT_3D('',#8320,#6614,#6615);
#5832=AXIS2_PLACEMENT_3D('',#8322,#6616,#6617);
#5833=AXIS2_PLACEMENT_3D('',#8323,#6618,#6619);
#5834=AXIS2_PLACEMENT_3D('',#8324,#6620,#6621);
#5835=AXIS2_PLACEMENT_3D('',#8326,#6622,#6623);
#5836=AXIS2_PLACEMENT_3D('',#8328,#6624,#6625);
#5837=AXIS2_PLACEMENT_3D('',#8329,#6626,#6627);
#5838=AXIS2_PLACEMENT_3D('',#8330,#6628,#6629);
#5839=AXIS2_PLACEMENT_3D('',#8332,#6630,#6631);
#5840=AXIS2_PLACEMENT_3D('',#8334,#6633,#6634);
#5841=AXIS2_PLACEMENT_3D('',#8336,#6635,#6636);
#5842=AXIS2_PLACEMENT_3D('',#8337,#6637,#6638);
#5843=AXIS2_PLACEMENT_3D('',#8338,#6639,#6640);
#5844=AXIS2_PLACEMENT_3D('',#8340,#6641,#6642);
#5845=AXIS2_PLACEMENT_3D('',#8342,#6643,#6644);
#5846=AXIS2_PLACEMENT_3D('',#8343,#6645,#6646);
#5847=AXIS2_PLACEMENT_3D('',#8344,#6647,#6648);
#5848=AXIS2_PLACEMENT_3D('',#8346,#6649,#6650);
#5849=AXIS2_PLACEMENT_3D('',#8348,#6652,#6653);
#5850=AXIS2_PLACEMENT_3D('',#8350,#6654,#6655);
#5851=AXIS2_PLACEMENT_3D('',#8351,#6656,#6657);
#5852=AXIS2_PLACEMENT_3D('',#8352,#6658,#6659);
#5853=AXIS2_PLACEMENT_3D('',#8354,#6660,#6661);
#5854=AXIS2_PLACEMENT_3D('',#8356,#6662,#6663);
#5855=AXIS2_PLACEMENT_3D('',#8357,#6664,#6665);
#5856=AXIS2_PLACEMENT_3D('',#8358,#6666,#6667);
#5857=AXIS2_PLACEMENT_3D('',#8360,#6668,#6669);
#5858=AXIS2_PLACEMENT_3D('',#8362,#6671,#6672);
#5859=AXIS2_PLACEMENT_3D('',#8363,#6673,#6674);
#5860=AXIS2_PLACEMENT_3D('',#8364,#6675,#6676);
#5861=AXIS2_PLACEMENT_3D('',#8365,#6677,#6678);
#5862=AXIS2_PLACEMENT_3D('',#8366,#6679,#6680);
#6373=DIRECTION('axis',(0.,0.,1.));
#6374=DIRECTION('refdir',(1.,0.,0.));
#6375=DIRECTION('center_axis',(-1.,-1.83697019872103E-16,0.));
#6376=DIRECTION('ref_axis',(1.83697019872103E-16,-1.,0.));
#6377=DIRECTION('center_axis',(-1.,-1.83697019872103E-16,0.));
#6378=DIRECTION('ref_axis',(1.83697019872103E-16,-1.,0.));
#6379=DIRECTION('',(-1.,-1.83697019872103E-16,0.));
#6380=DIRECTION('center_axis',(-1.,-1.83697019872103E-16,0.));
#6381=DIRECTION('ref_axis',(1.83697019872103E-16,-1.,0.));
#6382=DIRECTION('center_axis',(-1.,-1.83697019872103E-16,0.));
#6383=DIRECTION('ref_axis',(1.83697019872103E-16,-1.,0.));
#6384=DIRECTION('center_axis',(-1.,-1.83697019872103E-16,0.));
#6385=DIRECTION('ref_axis',(1.83697019872103E-16,-1.,0.));
#6386=DIRECTION('',(-1.,-1.83697019872103E-16,0.));
#6387=DIRECTION('center_axis',(-1.,-1.83697019872103E-16,0.));
#6388=DIRECTION('ref_axis',(1.83697019872103E-16,-1.,0.));
#6389=DIRECTION('center_axis',(-1.,-1.83697019872103E-16,0.));
#6390=DIRECTION('ref_axis',(1.83697019872103E-16,-1.,0.));
#6391=DIRECTION('center_axis',(-1.,-1.83697019872103E-16,0.));
#6392=DIRECTION('ref_axis',(1.83697019872103E-16,-1.,0.));
#6393=DIRECTION('center_axis',(-1.,-1.83697019872103E-16,0.));
#6394=DIRECTION('ref_axis',(1.83697019872103E-16,-1.,0.));
#6395=DIRECTION('',(-1.,-1.83697019872103E-16,0.));
#6396=DIRECTION('center_axis',(-1.,-1.83697019872103E-16,0.));
#6397=DIRECTION('ref_axis',(1.83697019872103E-16,-1.,0.));
#6398=DIRECTION('center_axis',(1.,1.83697019872103E-16,0.));
#6399=DIRECTION('ref_axis',(-1.83697019872103E-16,1.,0.));
#6400=DIRECTION('',(0.707106781186551,-0.707106781186544,-8.6595605623549E-17));
#6401=DIRECTION('center_axis',(-1.,-1.83697019872103E-16,0.));
#6402=DIRECTION('ref_axis',(1.83697019872103E-16,-1.,0.));
#6403=DIRECTION('center_axis',(-1.,-1.83697019872103E-16,0.));
#6404=DIRECTION('ref_axis',(1.85037170770859E-16,-1.,0.));
#6405=DIRECTION('center_axis',(-1.,-1.83697019872103E-16,0.));
#6406=DIRECTION('ref_axis',(1.83697019872103E-16,-1.,0.));
#6407=DIRECTION('center_axis',(2.24963967399279E-32,-1.22464679914735E-16,
-1.));
#6408=DIRECTION('ref_axis',(-1.85037170770859E-16,1.,-1.22464679914735E-16));
#6409=DIRECTION('center_axis',(-1.,-1.83697019872103E-16,0.));
#6410=DIRECTION('ref_axis',(1.83697019872103E-16,-1.,0.));
#6411=DIRECTION('center_axis',(-1.,-1.83697019872103E-16,0.));
#6412=DIRECTION('ref_axis',(1.83697019872103E-16,-1.,0.));
#6413=DIRECTION('center_axis',(-1.,-1.83697019872103E-16,0.));
#6414=DIRECTION('ref_axis',(1.83697019872103E-16,-1.,0.));
#6415=DIRECTION('',(1.,1.83697019872103E-16,0.));
#6416=DIRECTION('center_axis',(-1.,-1.83697019872103E-16,0.));
#6417=DIRECTION('ref_axis',(1.85037170770859E-16,-1.,0.));
#6418=DIRECTION('center_axis',(-1.,-1.83697019872103E-16,0.));
#6419=DIRECTION('ref_axis',(1.83697019872103E-16,-1.,0.));
#6420=DIRECTION('center_axis',(2.24963967399279E-32,-1.22464679914735E-16,
-1.));
#6421=DIRECTION('ref_axis',(-1.85037170770859E-16,1.,-1.22464679914735E-16));
#6422=DIRECTION('center_axis',(-1.,-1.83697019872103E-16,0.));
#6423=DIRECTION('ref_axis',(1.83697019872103E-16,-1.,0.));
#6424=DIRECTION('',(-0.707106781186551,0.707106781186544,-8.6595605623549E-17));
#6425=DIRECTION('center_axis',(-1.,-1.83697019872103E-16,0.));
#6426=DIRECTION('ref_axis',(1.83697019872103E-16,-1.,0.));
#6427=DIRECTION('center_axis',(1.,1.83697019872103E-16,0.));
#6428=DIRECTION('ref_axis',(-1.83697019872103E-16,1.,0.));
#6429=DIRECTION('center_axis',(-1.,-1.83697019872103E-16,0.));
#6430=DIRECTION('ref_axis',(1.83697019872103E-16,-1.,0.));
#6431=DIRECTION('center_axis',(1.,1.83697019872103E-16,0.));
#6432=DIRECTION('ref_axis',(-1.83697019872103E-16,1.,0.));
#6433=DIRECTION('center_axis',(-1.,-1.83697019872103E-16,0.));
#6434=DIRECTION('ref_axis',(1.83697019872103E-16,-1.,0.));
#6435=DIRECTION('center_axis',(1.,1.83697019872103E-16,0.));
#6436=DIRECTION('ref_axis',(-1.83697019872103E-16,1.,0.));
#6437=DIRECTION('center_axis',(-1.,-1.83697019872103E-16,0.));
#6438=DIRECTION('ref_axis',(1.83697019872103E-16,-1.,0.));
#6439=DIRECTION('',(-0.707106781186548,0.707106781186547,8.65956056235493E-17));
#6440=DIRECTION('center_axis',(-1.,-1.83697019872103E-16,0.));
#6441=DIRECTION('ref_axis',(1.83697019872103E-16,-1.,0.));
#6442=DIRECTION('center_axis',(-1.,-1.83697019872103E-16,0.));
#6443=DIRECTION('ref_axis',(1.83697019872103E-16,-1.,0.));
#6444=DIRECTION('center_axis',(-1.,-1.83697019872103E-16,0.));
#6445=DIRECTION('ref_axis',(1.83697019872103E-16,-1.,0.));
#6446=DIRECTION('',(1.,1.83697019872103E-16,0.));
#6447=DIRECTION('center_axis',(-1.,-1.83697019872103E-16,0.));
#6448=DIRECTION('ref_axis',(1.83697019872103E-16,-1.,0.));
#6449=DIRECTION('center_axis',(-1.,-1.83697019872103E-16,0.));
#6450=DIRECTION('ref_axis',(1.96129949112834E-16,-1.,0.));
#6451=DIRECTION('center_axis',(-2.24963967399279E-32,1.22464679914735E-16,
1.));
#6452=DIRECTION('ref_axis',(-1.63441624260695E-16,1.,-1.22464679914735E-16));
#6453=DIRECTION('center_axis',(-1.,-1.83697019872103E-16,0.));
#6454=DIRECTION('ref_axis',(1.83697019872103E-16,-1.,0.));
#6455=DIRECTION('center_axis',(-1.,-1.83697019872103E-16,0.));
#6456=DIRECTION('ref_axis',(1.83697019872103E-16,-1.,0.));
#6457=DIRECTION('center_axis',(-1.,-1.83697019872103E-16,0.));
#6458=DIRECTION('ref_axis',(1.83697019872103E-16,-1.,0.));
#6459=DIRECTION('',(1.,1.83697019872103E-16,0.));
#6460=DIRECTION('center_axis',(-1.,-1.83697019872103E-16,0.));
#6461=DIRECTION('ref_axis',(1.83697019872103E-16,-1.,0.));
#6462=DIRECTION('center_axis',(-1.,-1.83697019872103E-16,0.));
#6463=DIRECTION('ref_axis',(1.96129949112834E-16,-1.,0.));
#6464=DIRECTION('center_axis',(-1.,-1.83697019872103E-16,0.));
#6465=DIRECTION('ref_axis',(1.83697019872103E-16,-1.,0.));
#6466=DIRECTION('center_axis',(-2.24963967399279E-32,1.22464679914735E-16,
1.));
#6467=DIRECTION('ref_axis',(-1.63441624260695E-16,1.,-1.22464679914735E-16));
#6468=DIRECTION('center_axis',(-1.,-1.83697019872103E-16,0.));
#6469=DIRECTION('ref_axis',(1.83697019872103E-16,-1.,0.));
#6470=DIRECTION('center_axis',(-1.,-1.83697019872103E-16,0.));
#6471=DIRECTION('ref_axis',(1.83697019872103E-16,-1.,0.));
#6472=DIRECTION('',(1.,1.83697019872103E-16,0.));
#6473=DIRECTION('center_axis',(-1.,-1.83697019872103E-16,0.));
#6474=DIRECTION('ref_axis',(1.83697019872103E-16,-1.,0.));
#6475=DIRECTION('center_axis',(-1.,-1.83697019872103E-16,0.));
#6476=DIRECTION('ref_axis',(1.83697019872103E-16,-1.,0.));
#6477=DIRECTION('',(0.707106781186548,-0.707106781186547,8.65956056235493E-17));
#6478=DIRECTION('center_axis',(-1.,-1.83697019872103E-16,0.));
#6479=DIRECTION('ref_axis',(1.83697019872103E-16,-1.,0.));
#6480=DIRECTION('center_axis',(-1.,-1.83697019872103E-16,0.));
#6481=DIRECTION('ref_axis',(1.85037170770859E-16,-1.,0.));
#6482=DIRECTION('center_axis',(-1.,-1.83697019872103E-16,0.));
#6483=DIRECTION('ref_axis',(1.83697019872103E-16,-1.,0.));
#6484=DIRECTION('center_axis',(2.24963967399279E-32,-1.22464679914735E-16,
-1.));
#6485=DIRECTION('ref_axis',(-2.31296463463574E-16,1.,-1.22464679914735E-16));
#6486=DIRECTION('center_axis',(-1.,-1.83697019872103E-16,0.));
#6487=DIRECTION('ref_axis',(1.83697019872103E-16,-1.,0.));
#6488=DIRECTION('center_axis',(-1.,-1.83697019872103E-16,0.));
#6489=DIRECTION('ref_axis',(1.83697019872103E-16,-1.,0.));
#6490=DIRECTION('',(-1.,-1.83697019872103E-16,0.));
#6491=DIRECTION('center_axis',(-1.,-1.83697019872103E-16,0.));
#6492=DIRECTION('ref_axis',(1.83697019872103E-16,-1.,0.));
#6493=DIRECTION('center_axis',(-1.,-1.83697019872103E-16,0.));
#6494=DIRECTION('ref_axis',(1.85037170770859E-16,-1.,0.));
#6495=DIRECTION('center_axis',(2.24963967399279E-32,-1.22464679914735E-16,
-1.));
#6496=DIRECTION('ref_axis',(-2.31296463463574E-16,1.,-1.22464679914735E-16));
#6497=DIRECTION('center_axis',(-1.,-1.83697019872103E-16,0.));
#6498=DIRECTION('ref_axis',(1.83697019872103E-16,-1.,0.));
#6499=DIRECTION('center_axis',(-1.,-1.83697019872103E-16,0.));
#6500=DIRECTION('ref_axis',(1.83697019872103E-16,-1.,0.));
#6501=DIRECTION('center_axis',(-1.,-1.83697019872103E-16,0.));
#6502=DIRECTION('ref_axis',(1.83697019872103E-16,-1.,0.));
#6503=DIRECTION('center_axis',(1.,1.83697019872103E-16,0.));
#6504=DIRECTION('ref_axis',(-1.83697019872103E-16,1.,0.));
#6505=DIRECTION('center_axis',(1.,1.83697019872103E-16,0.));
#6506=DIRECTION('ref_axis',(-1.83697019872103E-16,1.,0.));
#6507=DIRECTION('center_axis',(-1.,-1.83697019872103E-16,0.));
#6508=DIRECTION('ref_axis',(1.83697019872103E-16,-1.,0.));
#6509=DIRECTION('center_axis',(-1.,-1.83697019872103E-16,0.));
#6510=DIRECTION('ref_axis',(1.83697019872103E-16,-1.,0.));
#6511=DIRECTION('',(-1.,-1.83697019872103E-16,0.));
#6512=DIRECTION('center_axis',(-1.,-1.83697019872103E-16,0.));
#6513=DIRECTION('ref_axis',(1.83697019872103E-16,-1.,0.));
#6514=DIRECTION('center_axis',(-1.,-1.83697019872103E-16,0.));
#6515=DIRECTION('ref_axis',(1.57361694361665E-16,-1.,0.));
#6516=DIRECTION('center_axis',(-1.,-1.83697019872103E-16,0.));
#6517=DIRECTION('ref_axis',(1.83697019872103E-16,-1.,0.));
#6518=DIRECTION('center_axis',(2.24963967399279E-32,-1.22464679914735E-16,
-1.));
#6519=DIRECTION('ref_axis',(-1.96702117952081E-16,1.,-1.22464679914735E-16));
#6520=DIRECTION('center_axis',(-1.,-1.83697019872103E-16,0.));
#6521=DIRECTION('ref_axis',(1.83697019872103E-16,-1.,0.));
#6522=DIRECTION('center_axis',(-1.,-1.83697019872103E-16,0.));
#6523=DIRECTION('ref_axis',(1.83697019872103E-16,-1.,0.));
#6524=DIRECTION('center_axis',(-1.,-1.83697019872103E-16,0.));
#6525=DIRECTION('ref_axis',(1.83697019872103E-16,-1.,0.));
#6526=DIRECTION('',(0.866025403784443,-0.499999999999992,6.12323399573667E-17));
#6527=DIRECTION('center_axis',(-1.,-1.83697019872103E-16,0.));
#6528=DIRECTION('ref_axis',(2.01689087919369E-16,-1.,0.));
#6529=DIRECTION('center_axis',(-1.,-1.83697019872103E-16,0.));
#6530=DIRECTION('ref_axis',(1.83697019872103E-16,-1.,0.));
#6531=DIRECTION('center_axis',(-2.24963967399279E-32,1.22464679914735E-16,
1.));
#6532=DIRECTION('ref_axis',(-1.89083519924408E-16,1.,-1.22464679914735E-16));
#6533=DIRECTION('center_axis',(-1.,-1.83697019872103E-16,0.));
#6534=DIRECTION('ref_axis',(1.88974131851091E-16,-1.,0.));
#6535=DIRECTION('center_axis',(-1.,-1.83697019872103E-16,0.));
#6536=DIRECTION('ref_axis',(1.83697019872103E-16,-1.,0.));
#6537=DIRECTION('center_axis',(-2.24963967399279E-32,1.22464679914735E-16,
1.));
#6538=DIRECTION('ref_axis',(-1.77163248610397E-16,1.,-1.22464679914735E-16));
#6539=DIRECTION('center_axis',(-1.,-1.83697019872103E-16,0.));
#6540=DIRECTION('ref_axis',(1.83697019872103E-16,-1.,0.));
#6541=DIRECTION('center_axis',(-1.,-1.83697019872103E-16,0.));
#6542=DIRECTION('ref_axis',(1.83697019872103E-16,-1.,0.));
#6543=DIRECTION('center_axis',(-1.,-1.83697019872103E-16,0.));
#6544=DIRECTION('ref_axis',(1.83697019872103E-16,-1.,0.));
#6545=DIRECTION('',(-0.500000000000007,0.866025403784435,-1.0605752387249E-16));
#6546=DIRECTION('center_axis',(-1.,-1.83697019872103E-16,0.));
#6547=DIRECTION('ref_axis',(1.91801449774277E-16,-1.,0.));
#6548=DIRECTION('center_axis',(-1.,-1.83697019872103E-16,0.));
#6549=DIRECTION('ref_axis',(1.83697019872103E-16,-1.,0.));
#6550=DIRECTION('center_axis',(-2.24963967399279E-32,1.22464679914735E-16,
1.));
#6551=DIRECTION('ref_axis',(-1.79813859163385E-16,1.,-1.22464679914735E-16));
#6552=DIRECTION('center_axis',(-1.,-1.83697019872103E-16,0.));
#6553=DIRECTION('ref_axis',(1.87747066251861E-16,-1.,0.));
#6554=DIRECTION('center_axis',(-1.,-1.83697019872103E-16,0.));
#6555=DIRECTION('ref_axis',(1.83697019872103E-16,-1.,0.));
#6556=DIRECTION('center_axis',(2.24963967399279E-32,-1.22464679914735E-16,
-1.));
#6557=DIRECTION('ref_axis',(-1.7601287461112E-16,1.,-1.22464679914735E-16));
#6558=DIRECTION('center_axis',(-1.,-1.83697019872103E-16,0.));
#6559=DIRECTION('ref_axis',(1.83697019872103E-16,-1.,0.));
#6560=DIRECTION('center_axis',(-1.,-1.83697019872103E-16,0.));
#6561=DIRECTION('ref_axis',(1.83697019872103E-16,-1.,0.));
#6562=DIRECTION('center_axis',(-1.,-1.83697019872103E-16,0.));
#6563=DIRECTION('ref_axis',(1.83697019872103E-16,-1.,0.));
#6564=DIRECTION('',(0.500000000000007,-0.866025403784435,1.0605752387249E-16));
#6565=DIRECTION('center_axis',(-1.,-1.83697019872103E-16,0.));
#6566=DIRECTION('ref_axis',(1.85037170770859E-16,-1.,0.));
#6567=DIRECTION('center_axis',(-1.,-1.83697019872103E-16,0.));
#6568=DIRECTION('ref_axis',(1.83697019872103E-16,-1.,0.));
#6569=DIRECTION('center_axis',(2.24963967399279E-32,-1.22464679914735E-16,
-1.));
#6570=DIRECTION('ref_axis',(-1.73472347597681E-16,1.,-1.22464679914735E-16));
#6571=DIRECTION('center_axis',(-1.,-1.83697019872103E-16,0.));
#6572=DIRECTION('ref_axis',(1.97210791246963E-16,-1.,0.));
#6573=DIRECTION('center_axis',(-1.,-1.83697019872103E-16,0.));
#6574=DIRECTION('ref_axis',(1.83697019872103E-16,-1.,0.));
#6575=DIRECTION('center_axis',(2.24963967399279E-32,-1.22464679914735E-16,
-1.));
#6576=DIRECTION('ref_axis',(-1.84885116794028E-16,1.,-1.22464679914735E-16));
#6577=DIRECTION('center_axis',(-1.,-1.83697019872103E-16,0.));
#6578=DIRECTION('ref_axis',(1.83697019872103E-16,-1.,0.));
#6579=DIRECTION('center_axis',(-1.,-1.83697019872103E-16,0.));
#6580=DIRECTION('ref_axis',(1.83697019872103E-16,-1.,0.));
#6581=DIRECTION('center_axis',(-1.,-1.83697019872103E-16,0.));
#6582=DIRECTION('ref_axis',(1.83697019872103E-16,-1.,0.));
#6583=DIRECTION('',(-0.866025403784443,0.499999999999992,-6.12323399573667E-17));
#6584=DIRECTION('center_axis',(1.,1.83697019872103E-16,0.));
#6585=DIRECTION('ref_axis',(-1.83697019872103E-16,1.,0.));
#6586=DIRECTION('center_axis',(1.,1.83697019872103E-16,0.));
#6587=DIRECTION('ref_axis',(-1.83697019872103E-16,1.,0.));
#6588=DIRECTION('center_axis',(-1.,-1.83697019872103E-16,0.));
#6589=DIRECTION('ref_axis',(1.83697019872103E-16,-1.,0.));
#6590=DIRECTION('center_axis',(1.,1.83697019872103E-16,0.));
#6591=DIRECTION('ref_axis',(-1.83697019872103E-16,1.,0.));
#6592=DIRECTION('center_axis',(1.,1.83697019872103E-16,0.));
#6593=DIRECTION('ref_axis',(-1.83697019872103E-16,1.,0.));
#6594=DIRECTION('center_axis',(1.,-1.83697019872103E-16,0.));
#6595=DIRECTION('ref_axis',(-1.83697019872103E-16,-1.,0.));
#6596=DIRECTION('center_axis',(-1.,1.83697019872103E-16,0.));
#6597=DIRECTION('ref_axis',(-1.83697019872103E-16,-1.,0.));
#6598=DIRECTION('',(1.,-1.83697019872103E-16,0.));
#6599=DIRECTION('center_axis',(-1.,1.83697019872103E-16,0.));
#6600=DIRECTION('ref_axis',(-1.83697019872103E-16,-1.,0.));
#6601=DIRECTION('center_axis',(1.,-1.83697019872103E-16,0.));
#6602=DIRECTION('ref_axis',(-1.57361694361665E-16,-1.,0.));
#6603=DIRECTION('center_axis',(-1.,1.83697019872103E-16,0.));
#6604=DIRECTION('ref_axis',(-1.83697019872103E-16,-1.,0.));
#6605=DIRECTION('center_axis',(-2.24963967399279E-32,-1.22464679914735E-16,
1.));
#6606=DIRECTION('ref_axis',(1.96702117952081E-16,1.,1.22464679914735E-16));
#6607=DIRECTION('center_axis',(-1.,1.83697019872103E-16,0.));
#6608=DIRECTION('ref_axis',(-1.83697019872103E-16,-1.,0.));
#6609=DIRECTION('center_axis',(1.,-1.83697019872103E-16,0.));
#6610=DIRECTION('ref_axis',(-1.83697019872103E-16,-1.,0.));
#6611=DIRECTION('center_axis',(-1.,1.83697019872103E-16,0.));
#6612=DIRECTION('ref_axis',(-1.83697019872103E-16,-1.,0.));
#6613=DIRECTION('',(-0.866025403784443,-0.499999999999992,-6.12323399573667E-17));
#6614=DIRECTION('center_axis',(1.,-1.83697019872103E-16,0.));
#6615=DIRECTION('ref_axis',(-2.01689087919369E-16,-1.,0.));
#6616=DIRECTION('center_axis',(-1.,1.83697019872103E-16,0.));
#6617=DIRECTION('ref_axis',(-1.83697019872103E-16,-1.,0.));
#6618=DIRECTION('center_axis',(2.24963967399279E-32,1.22464679914735E-16,
-1.));
#6619=DIRECTION('ref_axis',(1.89083519924408E-16,1.,1.22464679914735E-16));
#6620=DIRECTION('center_axis',(1.,-1.83697019872103E-16,0.));
#6621=DIRECTION('ref_axis',(-1.88974131851091E-16,-1.,0.));
#6622=DIRECTION('center_axis',(-1.,1.83697019872103E-16,0.));
#6623=DIRECTION('ref_axis',(-1.83697019872103E-16,-1.,0.));
#6624=DIRECTION('center_axis',(2.24963967399279E-32,1.22464679914735E-16,
-1.));
#6625=DIRECTION('ref_axis',(1.77163248610397E-16,1.,1.22464679914735E-16));
#6626=DIRECTION('center_axis',(-1.,1.83697019872103E-16,0.));
#6627=DIRECTION('ref_axis',(-1.83697019872103E-16,-1.,0.));
#6628=DIRECTION('center_axis',(1.,-1.83697019872103E-16,0.));
#6629=DIRECTION('ref_axis',(-1.83697019872103E-16,-1.,0.));
#6630=DIRECTION('center_axis',(-1.,1.83697019872103E-16,0.));
#6631=DIRECTION('ref_axis',(-1.83697019872103E-16,-1.,0.));
#6632=DIRECTION('',(0.500000000000007,0.866025403784435,1.0605752387249E-16));
#6633=DIRECTION('center_axis',(1.,-1.83697019872103E-16,0.));
#6634=DIRECTION('ref_axis',(-1.91801449774277E-16,-1.,0.));
#6635=DIRECTION('center_axis',(-1.,1.83697019872103E-16,0.));
#6636=DIRECTION('ref_axis',(-1.83697019872103E-16,-1.,0.));
#6637=DIRECTION('center_axis',(2.24963967399279E-32,1.22464679914735E-16,
-1.));
#6638=DIRECTION('ref_axis',(1.79813859163385E-16,1.,1.22464679914735E-16));
#6639=DIRECTION('center_axis',(1.,-1.83697019872103E-16,0.));
#6640=DIRECTION('ref_axis',(-1.87747066251861E-16,-1.,0.));
#6641=DIRECTION('center_axis',(-1.,1.83697019872103E-16,0.));
#6642=DIRECTION('ref_axis',(-1.83697019872103E-16,-1.,0.));
#6643=DIRECTION('center_axis',(-2.24963967399279E-32,-1.22464679914735E-16,
1.));
#6644=DIRECTION('ref_axis',(1.7601287461112E-16,1.,1.22464679914735E-16));
#6645=DIRECTION('center_axis',(-1.,1.83697019872103E-16,0.));
#6646=DIRECTION('ref_axis',(-1.83697019872103E-16,-1.,0.));
#6647=DIRECTION('center_axis',(1.,-1.83697019872103E-16,0.));
#6648=DIRECTION('ref_axis',(-1.83697019872103E-16,-1.,0.));
#6649=DIRECTION('center_axis',(-1.,1.83697019872103E-16,0.));
#6650=DIRECTION('ref_axis',(-1.83697019872103E-16,-1.,0.));
#6651=DIRECTION('',(-0.500000000000007,-0.866025403784435,-1.0605752387249E-16));
#6652=DIRECTION('center_axis',(1.,-1.83697019872103E-16,0.));
#6653=DIRECTION('ref_axis',(-1.85037170770859E-16,-1.,0.));
#6654=DIRECTION('center_axis',(-1.,1.83697019872103E-16,0.));
#6655=DIRECTION('ref_axis',(-1.83697019872103E-16,-1.,0.));
#6656=DIRECTION('center_axis',(-2.24963967399279E-32,-1.22464679914735E-16,
1.));
#6657=DIRECTION('ref_axis',(1.73472347597681E-16,1.,1.22464679914735E-16));
#6658=DIRECTION('center_axis',(1.,-1.83697019872103E-16,0.));
#6659=DIRECTION('ref_axis',(-1.97210791246963E-16,-1.,0.));
#6660=DIRECTION('center_axis',(-1.,1.83697019872103E-16,0.));
#6661=DIRECTION('ref_axis',(-1.83697019872103E-16,-1.,0.));
#6662=DIRECTION('center_axis',(-2.24963967399279E-32,-1.22464679914735E-16,
1.));
#6663=DIRECTION('ref_axis',(1.84885116794028E-16,1.,1.22464679914735E-16));
#6664=DIRECTION('center_axis',(-1.,1.83697019872103E-16,0.));
#6665=DIRECTION('ref_axis',(-1.83697019872103E-16,-1.,0.));
#6666=DIRECTION('center_axis',(1.,-1.83697019872103E-16,0.));
#6667=DIRECTION('ref_axis',(-1.83697019872103E-16,-1.,0.));
#6668=DIRECTION('center_axis',(-1.,1.83697019872103E-16,0.));
#6669=DIRECTION('ref_axis',(-1.83697019872103E-16,-1.,0.));
#6670=DIRECTION('',(0.866025403784443,0.499999999999992,6.12323399573667E-17));
#6671=DIRECTION('center_axis',(-1.,1.83697019872103E-16,0.));
#6672=DIRECTION('ref_axis',(1.83697019872103E-16,1.,0.));
#6673=DIRECTION('center_axis',(-1.,1.83697019872103E-16,0.));
#6674=DIRECTION('ref_axis',(1.83697019872103E-16,1.,0.));
#6675=DIRECTION('center_axis',(1.,-1.83697019872103E-16,0.));
#6676=DIRECTION('ref_axis',(-1.83697019872103E-16,-1.,0.));
#6677=DIRECTION('center_axis',(-1.,1.83697019872103E-16,0.));
#6678=DIRECTION('ref_axis',(1.83697019872103E-16,1.,0.));
#6679=DIRECTION('center_axis',(-1.,1.83697019872103E-16,0.));
#6680=DIRECTION('ref_axis',(1.83697019872103E-16,1.,0.));
#8140=CARTESIAN_POINT('',(0.,0.,0.));
#8141=CARTESIAN_POINT('Origin',(-1.8,0.,0.));
#8142=CARTESIAN_POINT('',(-1.7,4.8,-5.8783046359073E-16));
#8143=CARTESIAN_POINT('Origin',(-1.7,1.83697019872105E-17,0.));
#8144=CARTESIAN_POINT('',(-1.955,4.8,-5.8783046359073E-16));
#8145=CARTESIAN_POINT('',(-1.8,4.8,-5.87830463590729E-16));
#8146=CARTESIAN_POINT('Origin',(-1.955,-2.84730380801758E-17,0.));
#8147=CARTESIAN_POINT('Origin',(-1.8,0.,0.));
#8148=CARTESIAN_POINT('',(1.7,4.872,-5.96647920544591E-16));
#8149=CARTESIAN_POINT('Origin',(1.7,6.42939569552361E-16,0.));
#8150=CARTESIAN_POINT('',(-1.7,4.872,-5.96647920544591E-16));
#8151=CARTESIAN_POINT('',(-1.8,4.872,-5.96647920544591E-16));
#8152=CARTESIAN_POINT('Origin',(-1.7,1.83697019872105E-17,0.));
#8153=CARTESIAN_POINT('Origin',(-1.8,0.,0.));
#8154=CARTESIAN_POINT('',(1.955,-4.8,5.90585918888811E-16));
#8155=CARTESIAN_POINT('',(1.955,4.8,-5.87830463590729E-16));
#8156=CARTESIAN_POINT('Origin',(1.955,6.89782309619747E-16,0.));
#8157=CARTESIAN_POINT('Origin',(1.955,6.89782309619747E-16,0.));
#8158=CARTESIAN_POINT('',(1.7,4.8,-5.87830463590729E-16));
#8159=CARTESIAN_POINT('',(-1.8,4.8,-5.87830463590729E-16));
#8160=CARTESIAN_POINT('Origin',(1.7,6.42939569552361E-16,0.));
#8161=CARTESIAN_POINT('Origin',(1.955,6.89782309619747E-16,0.));
#8162=CARTESIAN_POINT('',(2.,-4.845,-5.93341374186893E-16));
#8163=CARTESIAN_POINT('',(1.955,-4.8,-5.87830463590729E-16));
#8164=CARTESIAN_POINT('Origin',(2.,6.98048675513991E-16,0.));
#8165=CARTESIAN_POINT('Origin',(1.8,8.67361737988404E-16,0.));
#8166=CARTESIAN_POINT('',(1.8,6.,-7.34788079488412E-16));
#8167=CARTESIAN_POINT('Origin',(1.8,6.61309271539571E-16,0.));
#8168=CARTESIAN_POINT('',(2.,5.8,-7.10295143505465E-16));
#8169=CARTESIAN_POINT('Origin',(1.8,5.8,-7.10295143505465E-16));
#8170=CARTESIAN_POINT('Origin',(2.,6.98048675513991E-16,0.));
#8171=CARTESIAN_POINT('Origin',(-1.8,0.,0.));
#8172=CARTESIAN_POINT('',(-1.8,6.,-7.34788079488412E-16));
#8173=CARTESIAN_POINT('Origin',(-1.8,2.02467570659351E-31,0.));
#8174=CARTESIAN_POINT('',(-1.8,6.,-7.34788079488412E-16));
#8175=CARTESIAN_POINT('Origin',(-1.8,0.,0.));
#8176=CARTESIAN_POINT('',(-2.,5.8,-7.10295143505465E-16));
#8177=CARTESIAN_POINT('Origin',(-2.,-3.67394039744204E-17,0.));
#8178=CARTESIAN_POINT('Origin',(-1.8,5.8,-7.10295143505465E-16));
#8179=CARTESIAN_POINT('Origin',(-2.,-3.67394039744204E-17,0.));
#8180=CARTESIAN_POINT('',(-2.,4.845,-5.93341374186893E-16));
#8181=CARTESIAN_POINT('',(-2.,4.845,-5.93341374186893E-16));
#8182=CARTESIAN_POINT('Origin',(-2.,-3.67394039744204E-17,0.));
#8183=CARTESIAN_POINT('Origin',(-2.,5.8,0.));
#8184=CARTESIAN_POINT('Origin',(2.,5.8,0.));
#8185=CARTESIAN_POINT('Origin',(1.7,4.8,0.));
#8186=CARTESIAN_POINT('Origin',(-1.7,4.8,0.));
#8187=CARTESIAN_POINT('Origin',(-1.955,-2.84730380801757E-17,0.));
#8188=CARTESIAN_POINT('',(-1.955,3.1184375,3.81898450271607E-16));
#8189=CARTESIAN_POINT('',(-1.955,-3.1184375,-3.81898450271607E-16));
#8190=CARTESIAN_POINT('Origin',(-1.955,-2.84730380801757E-17,0.));
#8191=CARTESIAN_POINT('',(-2.,-3.0734375,-3.76387539675444E-16));
#8192=CARTESIAN_POINT('',(-1.955,-3.1184375,-3.81898450271607E-16));
#8193=CARTESIAN_POINT('Origin',(-2.,-3.67394039744204E-17,0.));
#8194=CARTESIAN_POINT('Origin',(-1.955,-2.84730380801757E-17,0.));
#8195=CARTESIAN_POINT('Origin',(-1.8,0.,0.));
#8196=CARTESIAN_POINT('',(-1.7890625,3.1184375,-3.81898450271607E-16));
#8197=CARTESIAN_POINT('',(-1.8,3.1184375,-3.81898450271607E-16));
#8198=CARTESIAN_POINT('Origin',(-1.7890625,2.00918615485137E-18,0.));
#8199=CARTESIAN_POINT('Origin',(-1.7890625,0.,0.));
#8200=CARTESIAN_POINT('',(-1.6625,3.2,-3.91886975727153E-16));
#8201=CARTESIAN_POINT('Origin',(-1.7890625,3.25741379310345,-3.98918137522258E-16));
#8202=CARTESIAN_POINT('Origin',(-1.6625,2.52583402324144E-17,0.));
#8203=CARTESIAN_POINT('Origin',(-1.8,0.,0.));
#8204=CARTESIAN_POINT('',(-1.6625,3.272,-4.00704432681014E-16));
#8205=CARTESIAN_POINT('Origin',(-1.6625,2.52583402324144E-17,0.));
#8206=CARTESIAN_POINT('',(1.6625,3.272,-4.00704432681014E-16));
#8207=CARTESIAN_POINT('',(-1.8,3.272,-4.00704432681014E-16));
#8208=CARTESIAN_POINT('Origin',(1.6625,6.36050931307157E-16,0.));
#8209=CARTESIAN_POINT('Origin',(1.7890625,8.67361737988404E-16,0.));
#8210=CARTESIAN_POINT('',(1.6625,3.2,-3.91886975727153E-16));
#8211=CARTESIAN_POINT('Origin',(1.6625,6.36050931307157E-16,0.));
#8212=CARTESIAN_POINT('',(1.7890625,3.1184375,-3.81898450271607E-16));
#8213=CARTESIAN_POINT('Origin',(1.7890625,3.25741379310345,-3.98918137522258E-16));
#8214=CARTESIAN_POINT('Origin',(1.7890625,6.5930008538472E-16,0.));
#8215=CARTESIAN_POINT('Origin',(-1.8,0.,0.));
#8216=CARTESIAN_POINT('',(1.955,3.1184375,-3.81898450271607E-16));
#8217=CARTESIAN_POINT('',(-1.8,3.1184375,-3.81898450271607E-16));
#8218=CARTESIAN_POINT('Origin',(1.955,6.89782309619747E-16,0.));
#8219=CARTESIAN_POINT('Origin',(2.,6.98048675513991E-16,0.));
#8220=CARTESIAN_POINT('',(2.,3.0734375,-3.76387539675444E-16));
#8221=CARTESIAN_POINT('',(2.,3.0734375,-3.76387539675444E-16));
#8222=CARTESIAN_POINT('Origin',(2.,6.98048675513991E-16,0.));
#8223=CARTESIAN_POINT('Origin',(1.8,8.67361737988404E-16,0.));
#8224=CARTESIAN_POINT('',(2.,2.2,-2.69422295812418E-16));
#8225=CARTESIAN_POINT('Origin',(2.,6.98048675513991E-16,0.));
#8226=CARTESIAN_POINT('',(1.8,2.,-2.44929359829471E-16));
#8227=CARTESIAN_POINT('Origin',(1.8,2.2,-2.69422295812418E-16));
#8228=CARTESIAN_POINT('Origin',(1.8,6.61309271539571E-16,0.));
#8229=CARTESIAN_POINT('Origin',(-1.8,0.,0.));
#8230=CARTESIAN_POINT('',(-1.8,2.,-2.44929359829471E-16));
#8231=CARTESIAN_POINT('',(-1.8,2.,-2.44929359829471E-16));
#8232=CARTESIAN_POINT('Origin',(-1.8,1.86988015034452E-31,0.));
#8233=CARTESIAN_POINT('Origin',(-1.8,0.,0.));
#8234=CARTESIAN_POINT('',(-2.,2.2,-2.69422295812418E-16));
#8235=CARTESIAN_POINT('Origin',(-1.8,2.2,-2.69422295812418E-16));
#8236=CARTESIAN_POINT('Origin',(-2.,-3.67394039744205E-17,0.));
#8237=CARTESIAN_POINT('Origin',(2.,2.2,0.));
#8238=CARTESIAN_POINT('Origin',(1.6625,3.272,0.));
#8239=CARTESIAN_POINT('Origin',(-1.6625,3.2,0.));
#8240=CARTESIAN_POINT('Origin',(-2.,2.2,0.));
#8241=CARTESIAN_POINT('Origin',(-1.8,0.,0.));
#8242=CARTESIAN_POINT('',(1.95,3.2,-3.91886975727153E-16));
#8243=CARTESIAN_POINT('Origin',(1.95,6.88863824520387E-16,0.));
#8244=CARTESIAN_POINT('',(1.85,3.2,-3.91886975727153E-16));
#8245=CARTESIAN_POINT('',(-1.8,3.2,-3.91886975727153E-16));
#8246=CARTESIAN_POINT('Origin',(1.85,6.70494122533176E-16,0.));
#8247=CARTESIAN_POINT('Origin',(1.86,8.67361737988404E-16,0.));
#8248=CARTESIAN_POINT('',(1.905,4.22108058265378,-5.16933282449E-16));
#8249=CARTESIAN_POINT('Origin',(1.905,6.80597458626142E-16,0.));
#8250=CARTESIAN_POINT('',(1.95,4.14313829631318,-5.07388105300476E-16));
#8251=CARTESIAN_POINT('Origin',(1.86,4.14313829631318,-5.07388105300475E-16));
#8252=CARTESIAN_POINT('Origin',(1.95,6.88863824520387E-16,0.));
#8253=CARTESIAN_POINT('Origin',(1.65333333333334,6.34367041958329E-16,0.));
#8254=CARTESIAN_POINT('',(1.65333333333334,4.36638040039984,-5.3472737812094E-16));
#8255=CARTESIAN_POINT('Origin',(1.65333333333334,6.34367041958329E-16,0.));
#8256=CARTESIAN_POINT('',(1.65333333333334,4.36638040039984,-5.3472737812094E-16));
#8257=CARTESIAN_POINT('Origin',(1.66333333333334,8.67361737988404E-16,0.));
#8258=CARTESIAN_POINT('',(1.64333333333333,4.38370090847553,-5.3684852859839E-16));
#8259=CARTESIAN_POINT('Origin',(1.64333333333334,6.32530071759608E-16,0.));
#8260=CARTESIAN_POINT('Origin',(1.66333333333334,4.38370090847553,-5.3684852859839E-16));
#8261=CARTESIAN_POINT('Origin',(1.76333333333333,8.67361737988404E-16,0.));
#8262=CARTESIAN_POINT('',(1.86725638178747,4.64,-5.68236114804372E-16));
#8263=CARTESIAN_POINT('Origin',(1.86725638178747,6.73664068441309E-16,0.));
#8264=CARTESIAN_POINT('',(1.64333333333333,4.58,-5.60888234009488E-16));
#8265=CARTESIAN_POINT('Origin',(1.76333333333333,4.58,-5.60888234009488E-16));
#8266=CARTESIAN_POINT('Origin',(1.64333333333334,6.32530071759608E-16,0.));
#8267=CARTESIAN_POINT('Origin',(1.90725638178747,6.81011949236193E-16,0.));
#8268=CARTESIAN_POINT('',(1.90725638178747,4.57071796769724,-5.59751512894572E-16));
#8269=CARTESIAN_POINT('Origin',(1.90725638178747,6.81011949236193E-16,0.));
#8270=CARTESIAN_POINT('',(1.90725638178747,4.57071796769724,-5.59751512894572E-16));
#8271=CARTESIAN_POINT('Origin',(1.80333333333334,8.67361737988404E-16,0.));
#8272=CARTESIAN_POINT('',(1.80333333333334,4.39071796769724,-5.3770787050992E-16));
#8273=CARTESIAN_POINT('Origin',(1.80333333333334,6.61921594939145E-16,0.));
#8274=CARTESIAN_POINT('Origin',(1.80333333333334,4.51071796769724,-5.52403632099688E-16));
#8275=CARTESIAN_POINT('Origin',(1.80333333333334,8.67361737988404E-16,0.));
#8276=CARTESIAN_POINT('',(1.99385892216591,4.62071796769724,-5.65874746890309E-16));
#8277=CARTESIAN_POINT('Origin',(1.99385892216591,6.96920577817067E-16,0.));
#8278=CARTESIAN_POINT('',(1.80333333333334,4.29071796769724,-5.25461402518447E-16));
#8279=CARTESIAN_POINT('Origin',(1.80333333333334,4.51071796769724,-5.52403632099688E-16));
#8280=CARTESIAN_POINT('Origin',(1.80333333333334,6.61921594939145E-16,0.));
#8281=CARTESIAN_POINT('Origin',(1.99385892216591,6.96920577817067E-16,0.));
#8282=CARTESIAN_POINT('',(1.95385892216591,4.69,-5.74359348800109E-16));
#8283=CARTESIAN_POINT('Origin',(1.95385892216591,6.89572697022182E-16,0.));
#8284=CARTESIAN_POINT('',(1.99385892216591,4.62071796769724,-5.65874746890309E-16));
#8285=CARTESIAN_POINT('Origin',(1.76333333333333,8.67361737988404E-16,0.));
#8286=CARTESIAN_POINT('',(1.54333333333334,4.58,-5.60888234009488E-16));
#8287=CARTESIAN_POINT('Origin',(1.54333333333334,6.14160369772398E-16,0.));
#8288=CARTESIAN_POINT('Origin',(1.76333333333333,4.58,-5.60888234009488E-16));
#8289=CARTESIAN_POINT('Origin',(1.66333333333334,8.67361737988404E-16,0.));
#8290=CARTESIAN_POINT('',(1.60333333333334,4.27977786002139,-5.24121625733691E-16));
#8291=CARTESIAN_POINT('Origin',(1.60333333333334,6.25182190964724E-16,0.));
#8292=CARTESIAN_POINT('',(1.54333333333333,4.38370090847553,-5.3684852859839E-16));
#8293=CARTESIAN_POINT('Origin',(1.66333333333334,4.38370090847553,-5.3684852859839E-16));
#8294=CARTESIAN_POINT('Origin',(1.54333333333334,6.14160369772398E-16,0.));
#8295=CARTESIAN_POINT('Origin',(1.60333333333334,6.25182190964724E-16,0.));
#8296=CARTESIAN_POINT('',(1.85,4.13736479362129,-5.06681055141326E-16));
#8297=CARTESIAN_POINT('Origin',(1.85,6.70494122533176E-16,0.));
#8298=CARTESIAN_POINT('',(1.60333333333334,4.27977786002139,-5.2412162573369E-16));
#8299=CARTESIAN_POINT('Origin',(1.85,4.14313829631318,0.));
#8300=CARTESIAN_POINT('Origin',(1.54333333333334,4.58,0.));
#8301=CARTESIAN_POINT('Origin',(1.80333333333334,4.29071796769724,0.));
#8302=CARTESIAN_POINT('Origin',(1.64333333333334,4.58,0.));
#8303=CARTESIAN_POINT('Origin',(1.95,4.14313829631318,0.));
#8304=CARTESIAN_POINT('Origin',(1.8,0.,0.));
#8305=CARTESIAN_POINT('',(-1.95,3.2,3.91886975727153E-16));
#8306=CARTESIAN_POINT('Origin',(-1.95,6.88863824520387E-16,0.));
#8307=CARTESIAN_POINT('',(-1.85,3.2,3.91886975727153E-16));
#8308=CARTESIAN_POINT('',(1.8,3.2,3.91886975727153E-16));
#8309=CARTESIAN_POINT('Origin',(-1.85,6.70494122533176E-16,0.));
#8310=CARTESIAN_POINT('Origin',(-1.86,8.67361737988404E-16,0.));
#8311=CARTESIAN_POINT('',(-1.905,4.22108058265378,5.16933282449E-16));
#8312=CARTESIAN_POINT('Origin',(-1.905,6.80597458626142E-16,0.));
#8313=CARTESIAN_POINT('',(-1.95,4.14313829631318,5.07388105300476E-16));
#8314=CARTESIAN_POINT('Origin',(-1.86,4.14313829631318,5.07388105300475E-16));
#8315=CARTESIAN_POINT('Origin',(-1.95,6.88863824520387E-16,0.));
#8316=CARTESIAN_POINT('Origin',(-1.65333333333334,6.34367041958329E-16,
0.));
#8317=CARTESIAN_POINT('',(-1.65333333333334,4.36638040039984,5.3472737812094E-16));
#8318=CARTESIAN_POINT('Origin',(-1.65333333333334,6.34367041958329E-16,
0.));
#8319=CARTESIAN_POINT('',(-1.65333333333334,4.36638040039984,5.3472737812094E-16));
#8320=CARTESIAN_POINT('Origin',(-1.66333333333334,8.67361737988404E-16,
0.));
#8321=CARTESIAN_POINT('',(-1.64333333333333,4.38370090847553,5.3684852859839E-16));
#8322=CARTESIAN_POINT('Origin',(-1.64333333333334,6.32530071759608E-16,
0.));
#8323=CARTESIAN_POINT('Origin',(-1.66333333333334,4.38370090847553,5.3684852859839E-16));
#8324=CARTESIAN_POINT('Origin',(-1.76333333333333,8.67361737988404E-16,
0.));
#8325=CARTESIAN_POINT('',(-1.86725638178747,4.64,5.68236114804372E-16));
#8326=CARTESIAN_POINT('Origin',(-1.86725638178747,6.73664068441309E-16,
0.));
#8327=CARTESIAN_POINT('',(-1.64333333333333,4.58,5.60888234009488E-16));
#8328=CARTESIAN_POINT('Origin',(-1.76333333333333,4.58,5.60888234009488E-16));
#8329=CARTESIAN_POINT('Origin',(-1.64333333333334,6.32530071759608E-16,
0.));
#8330=CARTESIAN_POINT('Origin',(-1.90725638178747,6.81011949236193E-16,
0.));
#8331=CARTESIAN_POINT('',(-1.90725638178747,4.57071796769724,5.59751512894572E-16));
#8332=CARTESIAN_POINT('Origin',(-1.90725638178747,6.81011949236193E-16,
0.));
#8333=CARTESIAN_POINT('',(-1.90725638178747,4.57071796769724,5.59751512894572E-16));
#8334=CARTESIAN_POINT('Origin',(-1.80333333333334,8.67361737988404E-16,
0.));
#8335=CARTESIAN_POINT('',(-1.80333333333334,4.39071796769724,5.3770787050992E-16));
#8336=CARTESIAN_POINT('Origin',(-1.80333333333334,6.61921594939145E-16,
0.));
#8337=CARTESIAN_POINT('Origin',(-1.80333333333334,4.51071796769724,5.52403632099688E-16));
#8338=CARTESIAN_POINT('Origin',(-1.80333333333334,8.67361737988404E-16,
0.));
#8339=CARTESIAN_POINT('',(-1.99385892216591,4.62071796769724,5.65874746890309E-16));
#8340=CARTESIAN_POINT('Origin',(-1.99385892216591,6.96920577817067E-16,
0.));
#8341=CARTESIAN_POINT('',(-1.80333333333334,4.29071796769724,5.25461402518447E-16));
#8342=CARTESIAN_POINT('Origin',(-1.80333333333334,4.51071796769724,5.52403632099688E-16));
#8343=CARTESIAN_POINT('Origin',(-1.80333333333334,6.61921594939145E-16,
0.));
#8344=CARTESIAN_POINT('Origin',(-1.99385892216591,6.96920577817067E-16,
0.));
#8345=CARTESIAN_POINT('',(-1.95385892216591,4.69,5.74359348800109E-16));
#8346=CARTESIAN_POINT('Origin',(-1.95385892216591,6.89572697022182E-16,
0.));
#8347=CARTESIAN_POINT('',(-1.99385892216591,4.62071796769724,5.65874746890309E-16));
#8348=CARTESIAN_POINT('Origin',(-1.76333333333333,8.67361737988404E-16,
0.));
#8349=CARTESIAN_POINT('',(-1.54333333333334,4.58,5.60888234009488E-16));
#8350=CARTESIAN_POINT('Origin',(-1.54333333333334,6.14160369772398E-16,
0.));
#8351=CARTESIAN_POINT('Origin',(-1.76333333333333,4.58,5.60888234009488E-16));
#8352=CARTESIAN_POINT('Origin',(-1.66333333333334,8.67361737988404E-16,
0.));
#8353=CARTESIAN_POINT('',(-1.60333333333334,4.27977786002139,5.24121625733691E-16));
#8354=CARTESIAN_POINT('Origin',(-1.60333333333334,6.25182190964724E-16,
0.));
#8355=CARTESIAN_POINT('',(-1.54333333333333,4.38370090847553,5.3684852859839E-16));
#8356=CARTESIAN_POINT('Origin',(-1.66333333333334,4.38370090847553,5.3684852859839E-16));
#8357=CARTESIAN_POINT('Origin',(-1.54333333333334,6.14160369772398E-16,
0.));
#8358=CARTESIAN_POINT('Origin',(-1.60333333333334,6.25182190964724E-16,
0.));
#8359=CARTESIAN_POINT('',(-1.85,4.13736479362129,5.06681055141326E-16));
#8360=CARTESIAN_POINT('Origin',(-1.85,6.70494122533176E-16,0.));
#8361=CARTESIAN_POINT('',(-1.60333333333334,4.27977786002139,5.2412162573369E-16));
#8362=CARTESIAN_POINT('Origin',(-1.85,4.14313829631318,0.));
#8363=CARTESIAN_POINT('Origin',(-1.54333333333334,4.58,0.));
#8364=CARTESIAN_POINT('Origin',(-1.80333333333334,4.29071796769724,0.));
#8365=CARTESIAN_POINT('Origin',(-1.64333333333334,4.58,0.));
#8366=CARTESIAN_POINT('Origin',(-1.95,4.14313829631318,0.));
#9873=UNCERTAINTY_MEASURE_WITH_UNIT(LENGTH_MEASURE(0.01),#9892,
'DISTANCE_ACCURACY_VALUE',
'Maximum model space distance between geometric entities at asserted c
onnectivities');
#9881=UNCERTAINTY_MEASURE_WITH_UNIT(LENGTH_MEASURE(0.01),#9892,
'DISTANCE_ACCURACY_VALUE',
'Maximum model space distance between geometric entities at asserted c
onnectivities');
#9883=(
GEOMETRIC_REPRESENTATION_CONTEXT(3)
GLOBAL_UNCERTAINTY_ASSIGNED_CONTEXT((#9873))
GLOBAL_UNIT_ASSIGNED_CONTEXT((#9892,#9894,#9895))
REPRESENTATION_CONTEXT('','3D')
);
#9891=(
GEOMETRIC_REPRESENTATION_CONTEXT(3)
GLOBAL_UNCERTAINTY_ASSIGNED_CONTEXT((#9881))
GLOBAL_UNIT_ASSIGNED_CONTEXT((#9892,#9894,#9895))
REPRESENTATION_CONTEXT('','3D')
);
#9892=(
LENGTH_UNIT()
NAMED_UNIT(*)
SI_UNIT(.MILLI.,.METRE.)
);
#9894=(
NAMED_UNIT(*)
PLANE_ANGLE_UNIT()
SI_UNIT($,.RADIAN.)
);
#9895=(
NAMED_UNIT(*)
SI_UNIT($,.STERADIAN.)
SOLID_ANGLE_UNIT()
);
#9897=SHAPE_DEFINITION_REPRESENTATION(#9906,#9923);
#9906=PRODUCT_DEFINITION_SHAPE('',$,#9933);
#9923=SHAPE_REPRESENTATION('',(#5720),#9883);
#9931=PRODUCT_DEFINITION_CONTEXT('part definition',#9960,'design');
#9933=PRODUCT_DEFINITION(
'7804K102_Corrosion-Resistant 440C Stainless Steel Ball Bearing',
'Bearing_01',#9942,#9931);
#9942=PRODUCT_DEFINITION_FORMATION('',$,#9963);
#9960=APPLICATION_CONTEXT(
'Core Data for Automotive Mechanical Design Process');
#9961=PRODUCT_CONTEXT('part definition',#9960,'mechanical');
#9963=PRODUCT(
'7804K102_Corrosion-Resistant 440C Stainless Steel Ball Bearing',
'Bearing_01',$,(#9961));
#9972=PRESENTATION_STYLE_ASSIGNMENT((#9977));
#9977=SURFACE_STYLE_USAGE(.BOTH.,#9982);
#9982=SURFACE_SIDE_STYLE('',(#9987));
#9987=SURFACE_STYLE_FILL_AREA(#9992);
#9992=FILL_AREA_STYLE('Opaque(160,160,160)',(#9997));
#9997=FILL_AREA_STYLE_COLOUR('Opaque(160,160,160)',#10002);
#10002=COLOUR_RGB('Opaque(160,160,160)', 0.09019608, 0.27058824, 0.51372549);
ENDSEC;
END-ISO-10303-21;
